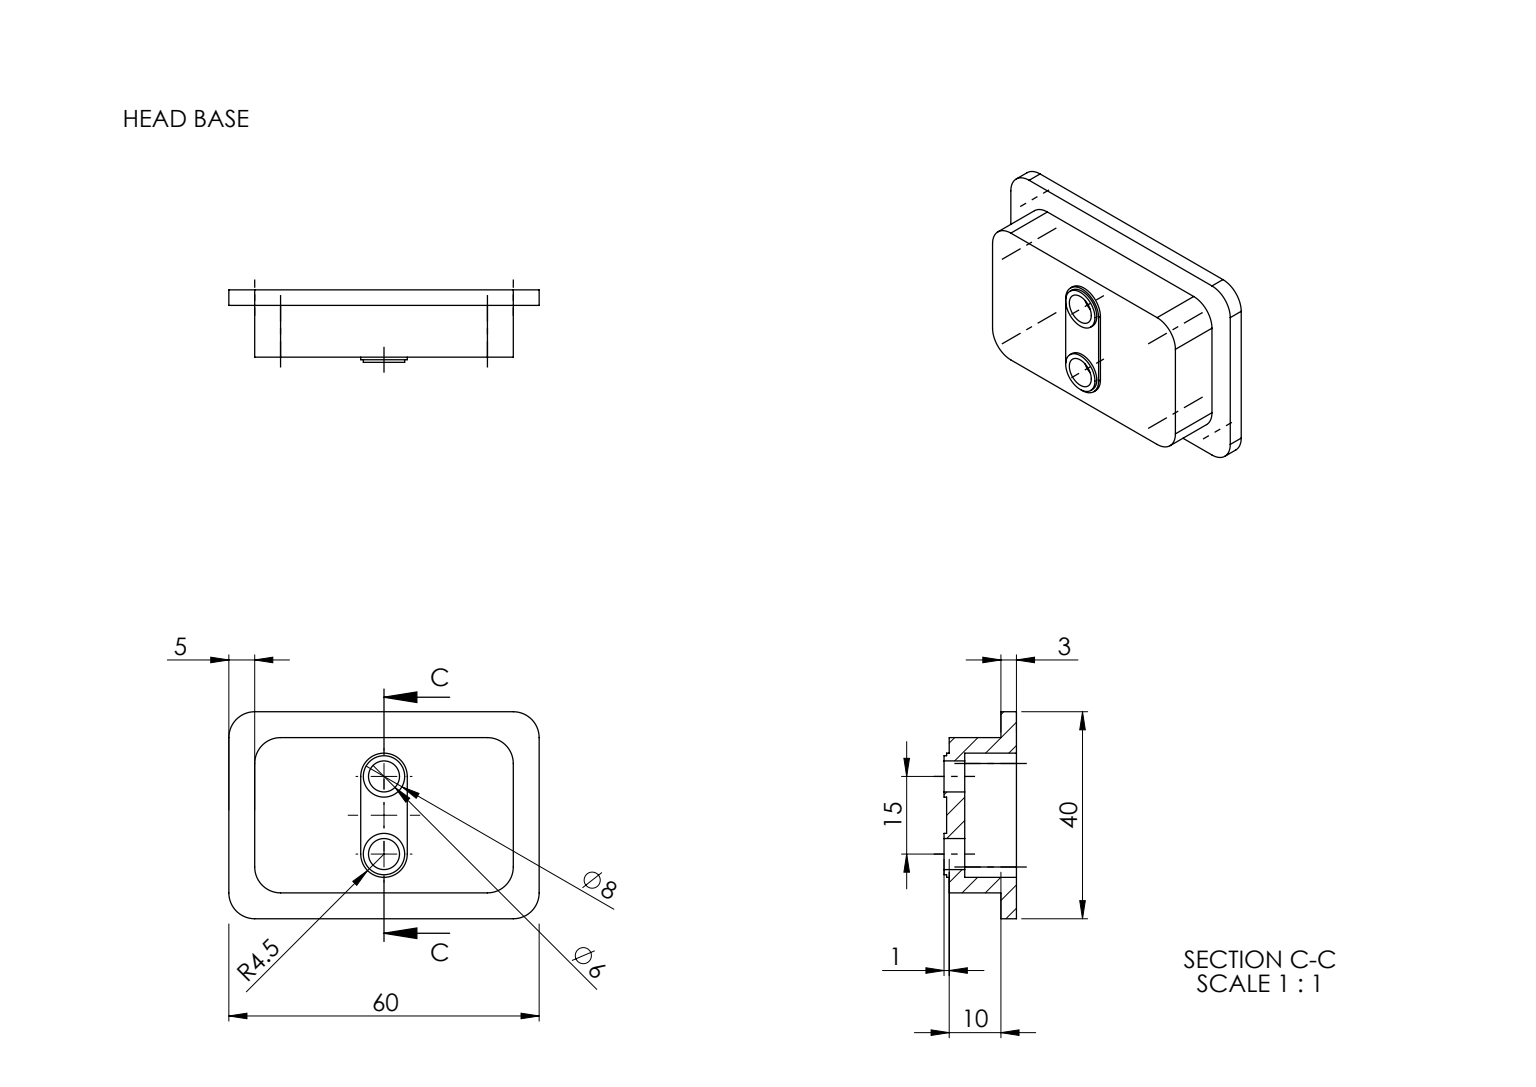
ISO-10303-21;
HEADER;
FILE_DESCRIPTION (('STEP AP214'),
    '1' );
FILE_NAME ('head base.step',
    '2026-10-05T05:16:24',
    ( '' ),
    ( '' ),
    'SwSTEP 2.0',
    'SolidWorks 2026',
    '' );
FILE_SCHEMA (( 'AUTOMOTIVE_DESIGN' ));
ENDSEC;

DATA;
#195=ORIENTED_EDGE ( 'NONE', *, *, #5496, .T. ) ;
#312=EDGE_CURVE ( 'NONE', #18504, #32170, #73011, .T. ) ;
#365=CARTESIAN_POINT ( 'NONE',  ( -19.99999999999996803, 12.00000000000000711, 13.00000000000000178 ) ) ;
#442=EDGE_CURVE ( 'NONE', #68729, #70011, #35447, .T. ) ;
#472=CARTESIAN_POINT ( 'NONE',  ( -19.99999999999996447, -15.00000000000000533, 13.00000000000000178 ) ) ;
#557=DIRECTION ( 'NONE',  ( -0.000000000000000000, -0.000000000000000000, 1.000000000000000000 ) ) ;
#647=ORIENTED_EDGE ( 'NONE', *, *, #5980, .F. ) ;
#855=FACE_OUTER_BOUND ( 'NONE', #52842, .T. ) ;
#984=EDGE_CURVE ( 'NONE', #16925, #51011, #66763, .T. ) ;
#1060=ORIENTED_EDGE ( 'NONE', *, *, #64186, .T. ) ;
#1108=VECTOR ( 'NONE', #67592, 1000.000000000000000 ) ;
#1176=CARTESIAN_POINT ( 'NONE',  ( -20.00000000000000355, 10.00000000000000711, 0.000000000000000000 ) ) ;
#1177=ORIENTED_EDGE ( 'NONE', *, *, #22871, .T. ) ;
#1205=EDGE_CURVE ( 'NONE', #18616, #63332, #75754, .T. ) ;
#1234=CARTESIAN_POINT ( 'NONE',  ( -30.00000000000000000, -15.00000000000000000, 0.000000000000000000 ) ) ;
#1306=EDGE_CURVE ( 'NONE', #63487, #26549, #52692, .T. ) ;
#1409=CARTESIAN_POINT ( 'NONE',  ( 1.653273178848927064E-15, -7.500000000000000000, 10.00000000000000178 ) ) ;
#1770=FACE_OUTER_BOUND ( 'NONE', #23896, .T. ) ;
#1802=EDGE_CURVE ( 'NONE', #18545, #32170, #34092, .T. ) ;
#2047=ORIENTED_EDGE ( 'NONE', *, *, #16725, .F. ) ;
#2074=EDGE_LOOP ( 'NONE', ( #21777, #5506, #55375, #74626, #78628, #49482, #5060, #5658 ) ) ;
#2087=EDGE_CURVE ( 'NONE', #19865, #25459, #46367, .T. ) ;
#2192=VERTEX_POINT ( 'NONE', #15248 ) ;
#2200=ORIENTED_EDGE ( 'NONE', *, *, #64434, .F. ) ;
#2202=DIRECTION ( 'NONE',  ( -1.000000000000000000, 0.000000000000000000, 0.000000000000000000 ) ) ;
#2315=VERTEX_POINT ( 'NONE', #64292 ) ;
#2378=DIRECTION ( 'NONE',  ( -1.000000000000000000, -0.000000000000000000, -0.000000000000000000 ) ) ;
#2534=CARTESIAN_POINT ( 'NONE',  ( 24.99999999999999645, -19.99999999999999645, 3.000000000000000000 ) ) ;
#2561=CARTESIAN_POINT ( 'NONE',  ( -2.939152317953646711E-15, 7.500000000000000000, 14.00000000000000178 ) ) ;
#2651=LINE ( 'NONE', #79222, #14432 ) ;
#2687=FACE_OUTER_BOUND ( 'NONE', #22273, .T. ) ;
#2987=DIRECTION ( 'NONE',  ( -0.000000000000000000, -0.000000000000000000, -1.000000000000000000 ) ) ;
#3039=ORIENTED_EDGE ( 'NONE', *, *, #49867, .T. ) ;
#3178=VECTOR ( 'NONE', #42643, 1000.000000000000000 ) ;
#3184=CARTESIAN_POINT ( 'NONE',  ( -4.000000000000002665, 7.500000000000000000, 14.00000000000000178 ) ) ;
#3289=ADVANCED_FACE ( 'NONE', ( #855 ), #21118, .F. ) ;
#3413=VERTEX_POINT ( 'NONE', #30098 ) ;
#3456=CARTESIAN_POINT ( 'NONE',  ( -24.99999999999999645, 20.00000000000000355, 3.000000000000000000 ) ) ;
#3577=LINE ( 'NONE', #17552, #29459 ) ;
#3768=EDGE_LOOP ( 'NONE', ( #32033, #51337, #64941, #21875 ) ) ;
#3841=FACE_OUTER_BOUND ( 'NONE', #46348, .T. ) ;
#4058=AXIS2_PLACEMENT_3D ( 'NONE', #29828, #76228, #28497 ) ;
#4063=EDGE_LOOP ( 'NONE', ( #83005, #56493, #12614, #77672 ) ) ;
#4204=DIRECTION ( 'NONE',  ( -1.000000000000000000, -2.602085213965214586E-16, 0.000000000000000000 ) ) ;
#4219=CIRCLE ( 'NONE', #9944, 2.000000000000001776 ) ;
#4406=AXIS2_PLACEMENT_3D ( 'NONE', #15425, #30695, #58160 ) ;
#4553=LINE ( 'NONE', #44629, #17255 ) ;
#4556=ORIENTED_EDGE ( 'NONE', *, *, #80069, .T. ) ;
#4604=CARTESIAN_POINT ( 'NONE',  ( 1.653273178848927064E-15, -7.500000000000000000, 14.00000000000000178 ) ) ;
#4629=FACE_OUTER_BOUND ( 'NONE', #4063, .T. ) ;
#4633=ADVANCED_FACE ( 'NONE', ( #24569 ), #63778, .T. ) ;
#4686=ADVANCED_FACE ( 'NONE', ( #25910 ), #17827, .F. ) ;
#4695=VERTEX_POINT ( 'NONE', #59692 ) ;
#4809=DIRECTION ( 'NONE',  ( 1.000000000000000000, 2.891205793294679312E-16, -0.000000000000000000 ) ) ;
#4928=AXIS2_PLACEMENT_3D ( 'NONE', #12936, #39980, #20576 ) ;
#4985=DIRECTION ( 'NONE',  ( -1.000000000000000000, 0.000000000000000000, 0.000000000000000000 ) ) ;
#5060=ORIENTED_EDGE ( 'NONE', *, *, #65557, .F. ) ;
#5101=LINE ( 'NONE', #66801, #28717 ) ;
#5110=VECTOR ( 'NONE', #83323, 1000.000000000000000 ) ;
#5172=VECTOR ( 'NONE', #59290, 1000.000000000000000 ) ;
#5413=EDGE_LOOP ( 'NONE', ( #8614, #19727 ) ) ;
#5496=EDGE_CURVE ( 'NONE', #18616, #70011, #21378, .T. ) ;
#5506=ORIENTED_EDGE ( 'NONE', *, *, #58155, .F. ) ;
#5519=ORIENTED_EDGE ( 'NONE', *, *, #46958, .F. ) ;
#5658=ORIENTED_EDGE ( 'NONE', *, *, #36655, .F. ) ;
#5674=( NAMED_UNIT ( * ) PLANE_ANGLE_UNIT ( ) SI_UNIT ( $, .RADIAN. ) );
#5765=CARTESIAN_POINT ( 'NONE',  ( 4.000000000000001776, -7.499999999999999112, 14.00000000000000178 ) ) ;
#5766=VERTEX_POINT ( 'NONE', #88001 ) ;
#5915=PRODUCT_CONTEXT ( 'NONE', #31413, 'mechanical' ) ;
#5969=DIRECTION ( 'NONE',  ( -1.000000000000000000, 0.000000000000000000, 0.000000000000000000 ) ) ;
#5980=EDGE_CURVE ( 'NONE', #81438, #38465, #26157, .T. ) ;
#6041=CARTESIAN_POINT ( 'NONE',  ( 22.00000000000000711, 9.999999999999971578, 10.00000000000000178 ) ) ;
#6065=CIRCLE ( 'NONE', #33378, 5.000000000000000888 ) ;
#6206=ORIENTED_EDGE ( 'NONE', *, *, #22249, .T. ) ;
#6220=ORIENTED_EDGE ( 'NONE', *, *, #1802, .T. ) ;
#6262=CARTESIAN_POINT ( 'NONE',  ( 25.00000000000000711, -9.999999999999957367, 3.000000000000000000 ) ) ;
#6281=LINE ( 'NONE', #81501, #58998 ) ;
#6523=CARTESIAN_POINT ( 'NONE',  ( 19.99999999999999289, -11.99999999999999467, 0.000000000000000000 ) ) ;
#6600=DIRECTION ( 'NONE',  ( -0.000000000000000000, -0.000000000000000000, 1.000000000000000000 ) ) ;
#6609=DIRECTION ( 'NONE',  ( 1.000000000000000000, 0.000000000000000000, 0.000000000000000000 ) ) ;
#6632=CARTESIAN_POINT ( 'NONE',  ( -25.00000000000000355, 9.999999999999971578, 3.000000000000000000 ) ) ;
#6641=ORIENTED_EDGE ( 'NONE', *, *, #16725, .T. ) ;
#6665=CIRCLE ( 'NONE', #57004, 5.000000000000000888 ) ;
#6846=EDGE_CURVE ( 'NONE', #66812, #61417, #24180, .T. ) ;
#6853=AXIS2_PLACEMENT_3D ( 'NONE', #39637, #81949, #32864 ) ;
#6906=DIRECTION ( 'NONE',  ( 1.734723475976812518E-16, -1.000000000000000000, 0.000000000000000000 ) ) ;
#6927=CARTESIAN_POINT ( 'NONE',  ( 20.00000000000000355, 10.00000000000000533, 13.00000000000000178 ) ) ;
#7173=DIRECTION ( 'NONE',  ( -0.000000000000000000, -0.000000000000000000, 1.000000000000000000 ) ) ;
#7184=CIRCLE ( 'NONE', #40303, 5.000000000000000888 ) ;
#7196=ORIENTED_EDGE ( 'NONE', *, *, #12757, .F. ) ;
#7303=EDGE_CURVE ( 'NONE', #16925, #38200, #58064, .T. ) ;
#7581=CARTESIAN_POINT ( 'NONE',  ( -2.939152317953646711E-15, 7.500000000000000000, 10.00000000000000178 ) ) ;
#7623=EDGE_CURVE ( 'NONE', #64470, #19590, #58845, .T. ) ;
#7645=EDGE_CURVE ( 'NONE', #69999, #32213, #86111, .T. ) ;
#7746=AXIS2_PLACEMENT_3D ( 'NONE', #88977, #53834, #14625 ) ;
#7760=FACE_OUTER_BOUND ( 'NONE', #35788, .T. ) ;
#7876=ORIENTED_EDGE ( 'NONE', *, *, #34261, .F. ) ;
#7893=ORIENTED_EDGE ( 'NONE', *, *, #21803, .F. ) ;
#7901=AXIS2_PLACEMENT_3D ( 'NONE', #17225, #51880, #38842 ) ;
#7983=ORIENTED_EDGE ( 'NONE', *, *, #56884, .F. ) ;
#8001=DIRECTION ( 'NONE',  ( -0.000000000000000000, -0.000000000000000000, -1.000000000000000000 ) ) ;
#8086=EDGE_CURVE ( 'NONE', #8684, #60639, #53111, .T. ) ;
#8216=ORIENTED_EDGE ( 'NONE', *, *, #51280, .F. ) ;
#8218=EDGE_CURVE ( 'NONE', #36898, #60372, #20437, .T. ) ;
#8277=LINE ( 'NONE', #56887, #35872 ) ;
#8309=VERTEX_POINT ( 'NONE', #69504 ) ;
#8320=DIRECTION ( 'NONE',  ( -0.000000000000000000, -0.000000000000000000, -1.000000000000000000 ) ) ;
#8330=ADVANCED_FACE ( 'NONE', ( #60368 ), #33352, .T. ) ;
#8402=VECTOR ( 'NONE', #71363, 1000.000000000000000 ) ;
#8408=DIRECTION ( 'NONE',  ( 1.000000000000000000, 0.000000000000000000, 0.000000000000000000 ) ) ;
#8537=AXIS2_PLACEMENT_3D ( 'NONE', #23795, #69789, #2202 ) ;
#8606=CIRCLE ( 'NONE', #58914, 4.500000000000001776 ) ;
#8614=ORIENTED_EDGE ( 'NONE', *, *, #76421, .F. ) ;
#8623=DIRECTION ( 'NONE',  ( 1.000000000000000000, 0.000000000000000000, 0.000000000000000000 ) ) ;
#8672=DIRECTION ( 'NONE',  ( 0.000000000000000000, 0.000000000000000000, 1.000000000000000000 ) ) ;
#8684=VERTEX_POINT ( 'NONE', #13111 ) ;
#8719=DIRECTION ( 'NONE',  ( 0.000000000000000000, 0.000000000000000000, 1.000000000000000000 ) ) ;
#8737=FACE_OUTER_BOUND ( 'NONE', #12896, .T. ) ;
#8784=AXIS2_PLACEMENT_3D ( 'NONE', #14973, #29817, #43326 ) ;
#8840=DIRECTION ( 'NONE',  ( -0.000000000000000000, -0.000000000000000000, -1.000000000000000000 ) ) ;
#8862=CARTESIAN_POINT ( 'NONE',  ( -30.00000000000000000, -15.00000000000000000, 3.000000000000000000 ) ) ;
#8964=EDGE_CURVE ( 'NONE', #8309, #60949, #86462, .T. ) ;
#9182=PRESENTATION_STYLE_ASSIGNMENT (( #42961 ) ) ;
#9211=CARTESIAN_POINT ( 'NONE',  ( -24.99999999999999645, -15.00000000000000000, 3.000000000000000000 ) ) ;
#9275=LINE ( 'NONE', #79051, #76492 ) ;
#9324=EDGE_CURVE ( 'NONE', #38200, #69999, #20864, .T. ) ;
#9651=VECTOR ( 'NONE', #77650, 1000.000000000000000 ) ;
#9660=EDGE_CURVE ( 'NONE', #30359, #38114, #86309, .T. ) ;
#9794=LINE ( 'NONE', #24640, #45704 ) ;
#9839=ADVANCED_FACE ( 'NONE', ( #2687, #15344 ), #42819, .T. ) ;
#9944=AXIS2_PLACEMENT_3D ( 'NONE', #70571, #83659, #76887 ) ;
#9994=AXIS2_PLACEMENT_3D ( 'NONE', #56497, #42983, #57818 ) ;
#10051=DIRECTION ( 'NONE',  ( 0.000000000000000000, 0.000000000000000000, 1.000000000000000000 ) ) ;
#10363=DIRECTION ( 'NONE',  ( -0.000000000000000000, -0.000000000000000000, -1.000000000000000000 ) ) ;
#10429=ORIENTED_EDGE ( 'NONE', *, *, #11533, .F. ) ;
#10541=AXIS2_PLACEMENT_3D ( 'NONE', #64258, #71913, #29614 ) ;
#10571=EDGE_CURVE ( 'NONE', #10700, #31320, #75066, .T. ) ;
#10596=CARTESIAN_POINT ( 'NONE',  ( 20.00000000000000711, -9.999999999999994671, 13.00000000000000178 ) ) ;
#10663=FILL_AREA_STYLE ('',( #72353 ) ) ;
#10700=VERTEX_POINT ( 'NONE', #85366 ) ;
#10748=ORIENTED_EDGE ( 'NONE', *, *, #18434, .T. ) ;
#10890=ORIENTED_EDGE ( 'NONE', *, *, #35603, .T. ) ;
#11062=ORIENTED_EDGE ( 'NONE', *, *, #24489, .F. ) ;
#11101=EDGE_LOOP ( 'NONE', ( #7876, #63098, #13245, #14650 ) ) ;
#11110=DIRECTION ( 'NONE',  ( 0.000000000000000000, 0.000000000000000000, 1.000000000000000000 ) ) ;
#11113=CARTESIAN_POINT ( 'NONE',  ( -2.939152317953646711E-15, 7.500000000000000000, 13.50000000000000178 ) ) ;
#11160=FACE_OUTER_BOUND ( 'NONE', #52351, .T. ) ;
#11256=LINE ( 'NONE', #59884, #79293 ) ;
#11358=PLANE ( 'NONE',  #7901 ) ;
#11403=ORIENTED_EDGE ( 'NONE', *, *, #67902, .T. ) ;
#11507=MECHANICAL_DESIGN_GEOMETRIC_PRESENTATION_REPRESENTATION('',(#14389),#21585);
#11533=EDGE_CURVE ( 'NONE', #68350, #38200, #11650, .T. ) ;
#11567=DIRECTION ( 'NONE',  ( 0.000000000000000000, 0.000000000000000000, 1.000000000000000000 ) ) ;
#11650=CIRCLE ( 'NONE', #83538, 2.000000000000001776 ) ;
#11703=EDGE_CURVE ( 'NONE', #32213, #60372, #13648, .T. ) ;
#11811=ORIENTED_EDGE ( 'NONE', *, *, #83550, .T. ) ;
#11889=ORIENTED_EDGE ( 'NONE', *, *, #9660, .T. ) ;
#11970=AXIS2_PLACEMENT_3D ( 'NONE', #40436, #48049, #8408 ) ;
#12354=PLANE ( 'NONE',  #13153 ) ;
#12436=CARTESIAN_POINT ( 'NONE',  ( -24.99999999999999645, 20.00000000000000355, 3.000000000000000000 ) ) ;
#12470=LINE ( 'NONE', #54330, #71773 ) ;
#12545=CARTESIAN_POINT ( 'NONE',  ( -24.99999999999999645, -19.99999999999999645, 0.000000000000000000 ) ) ;
#12614=ORIENTED_EDGE ( 'NONE', *, *, #23910, .F. ) ;
#12639=ORIENTED_EDGE ( 'NONE', *, *, #23910, .T. ) ;
#12694=ORIENTED_EDGE ( 'NONE', *, *, #19711, .T. ) ;
#12757=EDGE_CURVE ( 'NONE', #68985, #33215, #11256, .T. ) ;
#12830=ORIENTED_EDGE ( 'NONE', *, *, #84164, .F. ) ;
#12896=EDGE_LOOP ( 'NONE', ( #30436, #24948, #25039, #4556 ) ) ;
#12936=CARTESIAN_POINT ( 'NONE',  ( -24.99999999999999645, 15.00000000000000355, 3.000000000000000000 ) ) ;
#12944=FACE_OUTER_BOUND ( 'NONE', #69698, .T. ) ;
#13006=VECTOR ( 'NONE', #6600, 1000.000000000000000 ) ;
#13026=VECTOR ( 'NONE', #8001, 1000.000000000000000 ) ;
#13111=CARTESIAN_POINT ( 'NONE',  ( 24.99999999999999645, -19.99999999999999645, 0.000000000000000000 ) ) ;
#13129=CARTESIAN_POINT ( 'NONE',  ( -19.99999999999996803, 15.00000000000000711, 13.00000000000000178 ) ) ;
#13153=AXIS2_PLACEMENT_3D ( 'NONE', #59642, #53774, #87142 ) ;
#13231=VECTOR ( 'NONE', #19133, 1000.000000000000000 ) ;
#13245=ORIENTED_EDGE ( 'NONE', *, *, #13501, .T. ) ;
#13266=ORIENTED_EDGE ( 'NONE', *, *, #26362, .T. ) ;
#13271=CARTESIAN_POINT ( 'NONE',  ( 24.99999999999999645, -19.99999999999999645, 3.000000000000000000 ) ) ;
#13338=AXIS2_PLACEMENT_3D ( 'NONE', #365, #61609, #40908 ) ;
#13429=PLANE ( 'NONE',  #13338 ) ;
#13501=EDGE_CURVE ( 'NONE', #36898, #71705, #47720, .T. ) ;
#13528=VECTOR ( 'NONE', #71559, 1000.000000000000000 ) ;
#13638=CARTESIAN_POINT ( 'NONE',  ( 30.00000000000000000, 15.00000000000000355, 0.000000000000000000 ) ) ;
#13648=LINE ( 'NONE', #75789, #23148 ) ;
#13663=CARTESIAN_POINT ( 'NONE',  ( 3.000000000000001776, -7.500000000000000000, 0.000000000000000000 ) ) ;
#13752=LINE ( 'NONE', #53403, #13995 ) ;
#13768=CIRCLE ( 'NONE', #87166, 3.000000000000000444 ) ;
#13959=FACE_OUTER_BOUND ( 'NONE', #83885, .T. ) ;
#13995=VECTOR ( 'NONE', #20073, 1000.000000000000000 ) ;
#14051=ORIENTED_EDGE ( 'NONE', *, *, #5980, .T. ) ;
#14083=EDGE_CURVE ( 'NONE', #60639, #81205, #64753, .T. ) ;
#14126=EDGE_LOOP ( 'NONE', ( #30032, #47464, #76118, #83266 ) ) ;
#14164=AXIS2_PLACEMENT_3D ( 'NONE', #36806, #11110, #86352 ) ;
#14205=VERTEX_POINT ( 'NONE', #59789 ) ;
#14361=CARTESIAN_POINT ( 'NONE',  ( -22.00000000000000711, 9.999999999999971578, 0.000000000000000000 ) ) ;
#14389=STYLED_ITEM ( 'NONE', ( #9182 ), #73996 ) ;
#14432=VECTOR ( 'NONE', #60271, 1000.000000000000000 ) ;
#14572=ADVANCED_FACE ( 'NONE', ( #4629 ), #53249, .F. ) ;
#14604=EDGE_CURVE ( 'NONE', #51011, #17681, #57730, .T. ) ;
#14625=DIRECTION ( 'NONE',  ( 1.000000000000000000, 0.000000000000000000, -0.000000000000000000 ) ) ;
#14650=ORIENTED_EDGE ( 'NONE', *, *, #20454, .T. ) ;
#14708=DIRECTION ( 'NONE',  ( -0.000000000000000000, -0.000000000000000000, -1.000000000000000000 ) ) ;
#14744=ORIENTED_EDGE ( 'NONE', *, *, #70435, .T. ) ;
#14937=ORIENTED_EDGE ( 'NONE', *, *, #40107, .F. ) ;
#14973=CARTESIAN_POINT ( 'NONE',  ( 1.653273178848927064E-15, -7.500000000000000000, 14.00000000000000178 ) ) ;
#15066=ORIENTED_EDGE ( 'NONE', *, *, #60476, .F. ) ;
#15146=DIRECTION ( 'NONE',  ( 0.000000000000000000, 0.000000000000000000, 1.000000000000000000 ) ) ;
#15170=LINE ( 'NONE', #34986, #3178 ) ;
#15187=DIRECTION ( 'NONE',  ( -0.000000000000000000, -0.000000000000000000, -1.000000000000000000 ) ) ;
#15248=CARTESIAN_POINT ( 'NONE',  ( 19.99999999999996803, 12.00000000000000711, 10.00000000000000178 ) ) ;
#15344=FACE_BOUND ( 'NONE', #68935, .T. ) ;
#15377=AXIS2_PLACEMENT_3D ( 'NONE', #36820, #85019, #77366 ) ;
#15394=EDGE_LOOP ( 'NONE', ( #27022, #12830, #647, #52526 ) ) ;
#15419=FACE_BOUND ( 'NONE', #79429, .T. ) ;
#15425=CARTESIAN_POINT ( 'NONE',  ( 24.99999999999999645, 15.00000000000000355, 0.000000000000000000 ) ) ;
#15476=CARTESIAN_POINT ( 'NONE',  ( -24.99999999999999645, -15.00000000000000000, 0.000000000000000000 ) ) ;
#15490=SHAPE_REPRESENTATION_RELATIONSHIP ( 'NONE' , 'NONE' ,  #85713, #73996 ) ;
#15496=CARTESIAN_POINT ( 'NONE',  ( 1.653273178848927064E-15, -7.500000000000000000, 10.00000000000000178 ) ) ;
#15556=AXIS2_PLACEMENT_3D ( 'NONE', #57893, #17359, #70974 ) ;
#15637=VECTOR ( 'NONE', #45329, 1000.000000000000000 ) ;
#15638=ORIENTED_EDGE ( 'NONE', *, *, #83550, .F. ) ;
#15649=VERTEX_POINT ( 'NONE', #21728 ) ;
#15667=LINE ( 'NONE', #43137, #86476 ) ;
#15953=VECTOR ( 'NONE', #78730, 1000.000000000000000 ) ;
#16150=ORIENTED_EDGE ( 'NONE', *, *, #36183, .T. ) ;
#16324=CARTESIAN_POINT ( 'NONE',  ( 22.00000000000000711, 9.999999999999991118, 10.00000000000000178 ) ) ;
#16369=ORIENTED_EDGE ( 'NONE', *, *, #81297, .F. ) ;
#16389=PLANE ( 'NONE',  #38761 ) ;
#16399=ORIENTED_EDGE ( 'NONE', *, *, #78408, .F. ) ;
#16438=LINE ( 'NONE', #43907, #32432 ) ;
#16487=DIRECTION ( 'NONE',  ( -0.000000000000000000, -0.000000000000000000, -1.000000000000000000 ) ) ;
#16528=DIRECTION ( 'NONE',  ( 1.000000000000000000, 0.000000000000000000, 0.000000000000000000 ) ) ;
#16641=DIRECTION ( 'NONE',  ( 0.000000000000000000, 0.000000000000000000, 1.000000000000000000 ) ) ;
#16725=EDGE_CURVE ( 'NONE', #31293, #17102, #6065, .T. ) ;
#16783=DIRECTION ( 'NONE',  ( -1.000000000000000000, 0.000000000000000000, 0.000000000000000000 ) ) ;
#16805=VECTOR ( 'NONE', #67005, 1000.000000000000000 ) ;
#16889=VECTOR ( 'NONE', #87328, 1000.000000000000000 ) ;
#16900=DIRECTION ( 'NONE',  ( 1.000000000000000000, 0.000000000000000000, 0.000000000000000000 ) ) ;
#16925=VERTEX_POINT ( 'NONE', #23400 ) ;
#17037=ADVANCED_FACE ( 'NONE', ( #71148 ), #36917, .T. ) ;
#17051=VERTEX_POINT ( 'NONE', #34162 ) ;
#17093=EDGE_LOOP ( 'NONE', ( #83307, #21231, #88931, #17741 ) ) ;
#17102=VERTEX_POINT ( 'NONE', #6262 ) ;
#17111=CARTESIAN_POINT ( 'NONE',  ( -30.00000000000000000, 15.00000000000000355, 3.000000000000000000 ) ) ;
#17223=CARTESIAN_POINT ( 'NONE',  ( 1.653273178848927064E-15, -7.500000000000000000, 14.00000000000000178 ) ) ;
#17225=CARTESIAN_POINT ( 'NONE',  ( 4.499999999999999112, 7.500000000000002665, 13.50000000000000178 ) ) ;
#17229=DIRECTION ( 'NONE',  ( -1.000000000000000000, 0.000000000000000000, 0.000000000000000000 ) ) ;
#17255=VECTOR ( 'NONE', #24817, 1000.000000000000000 ) ;
#17344=CARTESIAN_POINT ( 'NONE',  ( -20.00000000000000355, -10.00000000000000533, 13.00000000000000178 ) ) ;
#17359=DIRECTION ( 'NONE',  ( -0.000000000000000000, -0.000000000000000000, -1.000000000000000000 ) ) ;
#17388=CIRCLE ( 'NONE', #46147, 5.000000000000000888 ) ;
#17524=FACE_BOUND ( 'NONE', #79964, .T. ) ;
#17552=CARTESIAN_POINT ( 'NONE',  ( 4.499999999999999112, 7.500000000000002665, 13.50000000000000178 ) ) ;
#17662=CARTESIAN_POINT ( 'NONE',  ( -30.00000000000000000, 15.00000000000000355, 3.000000000000000000 ) ) ;
#17681=VERTEX_POINT ( 'NONE', #65063 ) ;
#17741=ORIENTED_EDGE ( 'NONE', *, *, #21803, .T. ) ;
#17827=PLANE ( 'NONE',  #28511 ) ;
#17868=DIRECTION ( 'NONE',  ( 0.000000000000000000, 0.000000000000000000, 1.000000000000000000 ) ) ;
#17953=EDGE_LOOP ( 'NONE', ( #74100, #62548, #41992, #41745 ) ) ;
#17976=ORIENTED_EDGE ( 'NONE', *, *, #44356, .F. ) ;
#18066=EDGE_CURVE ( 'NONE', #40270, #61417, #25208, .T. ) ;
#18115=CARTESIAN_POINT ( 'NONE',  ( 19.99999999999999289, -11.99999999999999467, 10.00000000000000178 ) ) ;
#18149=CARTESIAN_POINT ( 'NONE',  ( 30.00000000000000000, -15.00000000000000000, 3.000000000000000000 ) ) ;
#18192=DIRECTION ( 'NONE',  ( 0.000000000000000000, 0.000000000000000000, 1.000000000000000000 ) ) ;
#18434=EDGE_CURVE ( 'NONE', #73496, #15649, #31557, .T. ) ;
#18466=EDGE_CURVE ( 'NONE', #59616, #19865, #46490, .T. ) ;
#18504=VERTEX_POINT ( 'NONE', #61566 ) ;
#18530=EDGE_CURVE ( 'NONE', #22067, #22580, #49391, .T. ) ;
#18545=VERTEX_POINT ( 'NONE', #48941 ) ;
#18616=VERTEX_POINT ( 'NONE', #57021 ) ;
#18653=LINE ( 'NONE', #59620, #76335 ) ;
#18674=FACE_OUTER_BOUND ( 'NONE', #2074, .T. ) ;
#18826=VERTEX_POINT ( 'NONE', #19157 ) ;
#18855=PLANE ( 'NONE',  #26581 ) ;
#18919=DIRECTION ( 'NONE',  ( -2.891205793294678326E-16, 1.000000000000000000, -0.000000000000000000 ) ) ;
#19056=ORIENTED_EDGE ( 'NONE', *, *, #26362, .F. ) ;
#19133=DIRECTION ( 'NONE',  ( -0.000000000000000000, -0.000000000000000000, -1.000000000000000000 ) ) ;
#19157=CARTESIAN_POINT ( 'NONE',  ( 30.00000000000000000, -15.00000000000000000, 3.000000000000000000 ) ) ;
#19175=EDGE_LOOP ( 'NONE', ( #34540, #16399, #80837, #56876 ) ) ;
#19177=ORIENTED_EDGE ( 'NONE', *, *, #75759, .T. ) ;
#19407=CIRCLE ( 'NONE', #88419, 3.000000000000000000 ) ;
#19474=DIRECTION ( 'NONE',  ( -0.000000000000000000, -0.000000000000000000, -1.000000000000000000 ) ) ;
#19503=FACE_OUTER_BOUND ( 'NONE', #73049, .T. ) ;
#19558=ORIENTED_EDGE ( 'NONE', *, *, #38282, .T. ) ;
#19590=VERTEX_POINT ( 'NONE', #36443 ) ;
#19606=FACE_OUTER_BOUND ( 'NONE', #49192, .T. ) ;
#19664=DIRECTION ( 'NONE',  ( 0.000000000000000000, 1.000000000000000000, 0.000000000000000000 ) ) ;
#19711=EDGE_CURVE ( 'NONE', #4695, #17051, #78748, .T. ) ;
#19727=ORIENTED_EDGE ( 'NONE', *, *, #36136, .F. ) ;
#19757=CARTESIAN_POINT ( 'NONE',  ( -24.99999999999999645, -19.99999999999999645, 3.000000000000000000 ) ) ;
#19865=VERTEX_POINT ( 'NONE', #5765 ) ;
#19892=ORIENTED_EDGE ( 'NONE', *, *, #42792, .T. ) ;
#19919=ORIENTED_EDGE ( 'NONE', *, *, #9324, .T. ) ;
#19944=ORIENTED_EDGE ( 'NONE', *, *, #62373, .F. ) ;
#20073=DIRECTION ( 'NONE',  ( -0.000000000000000000, -0.000000000000000000, -1.000000000000000000 ) ) ;
#20238=CIRCLE ( 'NONE', #4406, 5.000000000000000888 ) ;
#20400=VERTEX_POINT ( 'NONE', #31119 ) ;
#20413=DIRECTION ( 'NONE',  ( 0.000000000000000000, 0.000000000000000000, 1.000000000000000000 ) ) ;
#20437=LINE ( 'NONE', #40720, #48737 ) ;
#20454=EDGE_CURVE ( 'NONE', #71705, #22195, #74345, .T. ) ;
#20468=ORIENTED_EDGE ( 'NONE', *, *, #29865, .T. ) ;
#20576=DIRECTION ( 'NONE',  ( -1.000000000000000000, 0.000000000000000000, 0.000000000000000000 ) ) ;
#20587=ORIENTED_EDGE ( 'NONE', *, *, #46958, .T. ) ;
#20594=AXIS2_PLACEMENT_3D ( 'NONE', #56188, #17868, #39480 ) ;
#20864=LINE ( 'NONE', #34378, #48810 ) ;
#20928=FACE_BOUND ( 'NONE', #69239, .T. ) ;
#21028=EDGE_LOOP ( 'NONE', ( #31715, #28055, #61276, #11403 ) ) ;
#21031=CARTESIAN_POINT ( 'NONE',  ( -2.939152317953646711E-15, 7.500000000000000000, 14.00000000000000178 ) ) ;
#21077=DIRECTION ( 'NONE',  ( 1.000000000000000000, 0.000000000000000000, 0.000000000000000000 ) ) ;
#21118=CYLINDRICAL_SURFACE ( 'NONE', #68762, 3.000000000000000444 ) ;
#21231=ORIENTED_EDGE ( 'NONE', *, *, #80069, .F. ) ;
#21358=ORIENTED_EDGE ( 'NONE', *, *, #54212, .T. ) ;
#21371=ORIENTED_EDGE ( 'NONE', *, *, #8964, .T. ) ;
#21378=LINE ( 'NONE', #50161, #9651 ) ;
#21386=AXIS2_PLACEMENT_3D ( 'NONE', #8862, #56154, #63348 ) ;
#21552=AXIS2_PLACEMENT_3D ( 'NONE', #74381, #72595, #46464 ) ;
#21585=( GEOMETRIC_REPRESENTATION_CONTEXT ( 3 ) GLOBAL_UNCERTAINTY_ASSIGNED_CONTEXT ( ( #23001 ) ) GLOBAL_UNIT_ASSIGNED_CONTEXT ( ( #49270, #56469, #71296 ) ) REPRESENTATION_CONTEXT ( 'NONE', 'WORKASPACE' ) );
#21708=ORIENTED_EDGE ( 'NONE', *, *, #36136, .T. ) ;
#21728=CARTESIAN_POINT ( 'NONE',  ( 2.999999999999997335, 7.500000000000000000, 14.00000000000000178 ) ) ;
#21737=CARTESIAN_POINT ( 'NONE',  ( -25.00000000000000355, 9.999999999999971578, 3.000000000000000000 ) ) ;
#21777=ORIENTED_EDGE ( 'NONE', *, *, #13501, .F. ) ;
#21803=EDGE_CURVE ( 'NONE', #17681, #32213, #23708, .T. ) ;
#21824=VECTOR ( 'NONE', #56952, 1000.000000000000000 ) ;
#21827=CYLINDRICAL_SURFACE ( 'NONE', #68239, 5.000000000000000888 ) ;
#21857=CARTESIAN_POINT ( 'NONE',  ( -25.00000000000000355, 9.999999999999971578, 13.00000000000000178 ) ) ;
#21875=ORIENTED_EDGE ( 'NONE', *, *, #41723, .T. ) ;
#21950=ORIENTED_EDGE ( 'NONE', *, *, #22509, .F. ) ;
#21964=FACE_BOUND ( 'NONE', #79199, .T. ) ;
#22067=VERTEX_POINT ( 'NONE', #21737 ) ;
#22195=VERTEX_POINT ( 'NONE', #23937 ) ;
#22215=ORIENTED_EDGE ( 'NONE', *, *, #77394, .T. ) ;
#22249=EDGE_CURVE ( 'NONE', #32170, #79550, #81574, .T. ) ;
#22263=ADVANCED_FACE ( 'NONE', ( #32938 ), #60844, .F. ) ;
#22273=EDGE_LOOP ( 'NONE', ( #11062, #19944, #52099, #21950, #16369, #27894, #86581, #74895 ) ) ;
#22401=PLANE ( 'NONE',  #59441 ) ;
#22498=LINE ( 'NONE', #58047, #13528 ) ;
#22509=EDGE_CURVE ( 'NONE', #50943, #66812, #86912, .T. ) ;
#22580=VERTEX_POINT ( 'NONE', #39157 ) ;
#22694=CARTESIAN_POINT ( 'NONE',  ( 19.99999999999997158, -14.99999999999999467, 3.000000000000000000 ) ) ;
#22697=VECTOR ( 'NONE', #68168, 1000.000000000000000 ) ;
#22744=LINE ( 'NONE', #50204, #56420 ) ;
#22769=VECTOR ( 'NONE', #45437, 1000.000000000000000 ) ;
#22857=DIRECTION ( 'NONE',  ( 1.000000000000000000, 2.602085213965214586E-16, 0.000000000000000000 ) ) ;
#22863=VECTOR ( 'NONE', #15187, 1000.000000000000000 ) ;
#22871=EDGE_CURVE ( 'NONE', #85628, #8309, #8606, .T. ) ;
#22894=CARTESIAN_POINT ( 'NONE',  ( 30.00000000000000000, -15.00000000000000000, 0.000000000000000000 ) ) ;
#23001=UNCERTAINTY_MEASURE_WITH_UNIT (LENGTH_MEASURE( 1.000000000000000082E-05 ), #49270, 'distance_accuracy_value', 'NONE');
#23051=PRODUCT_DEFINITION_CONTEXT ( 'detailed design', #88395, 'design' ) ;
#23148=VECTOR ( 'NONE', #33484, 1000.000000000000000 ) ;
#23274=EDGE_CURVE ( 'NONE', #79550, #22067, #7184, .T. ) ;
#23400=CARTESIAN_POINT ( 'NONE',  ( -22.00000000000000711, 9.999999999999971578, 10.00000000000000178 ) ) ;
#23427=MECHANICAL_DESIGN_GEOMETRIC_PRESENTATION_REPRESENTATION('',(#63737),#55130);
#23608=CARTESIAN_POINT ( 'NONE',  ( 30.00000000000000000, 15.00000000000000355, 3.000000000000000000 ) ) ;
#23653=DIRECTION ( 'NONE',  ( -1.000000000000000000, 0.000000000000000000, 0.000000000000000000 ) ) ;
#23655=CARTESIAN_POINT ( 'NONE',  ( -22.00000000000000355, -10.00000000000000533, 0.000000000000000000 ) ) ;
#23708=LINE ( 'NONE', #36794, #68495 ) ;
#23733=VECTOR ( 'NONE', #34844, 1000.000000000000000 ) ;
#23749=DIRECTION ( 'NONE',  ( -1.734723475976813504E-16, 1.000000000000000000, 0.000000000000000000 ) ) ;
#23795=CARTESIAN_POINT ( 'NONE',  ( -2.939152317953646711E-15, 7.500000000000000000, 14.00000000000000178 ) ) ;
#23800=ORIENTED_EDGE ( 'NONE', *, *, #7645, .T. ) ;
#23896=EDGE_LOOP ( 'NONE', ( #31891, #88365, #42732, #62617 ) ) ;
#23910=EDGE_CURVE ( 'NONE', #18826, #84614, #40396, .T. ) ;
#23923=ORIENTED_EDGE ( 'NONE', *, *, #22509, .T. ) ;
#23924=VECTOR ( 'NONE', #87504, 1000.000000000000000 ) ;
#23937=CARTESIAN_POINT ( 'NONE',  ( 22.00000000000001066, -9.999999999999957367, 0.000000000000000000 ) ) ;
#23952=EDGE_LOOP ( 'NONE', ( #11889, #71790 ) ) ;
#24007=ORIENTED_EDGE ( 'NONE', *, *, #27409, .T. ) ;
#24032=CARTESIAN_POINT ( 'NONE',  ( -3.999999999999998224, -7.500000000000000000, 14.00000000000000178 ) ) ;
#24149=ADVANCED_FACE ( 'NONE', ( #37163 ), #30415, .F. ) ;
#24180=CIRCLE ( 'NONE', #4058, 5.000000000000000888 ) ;
#24197=PLANE ( 'NONE',  #45421 ) ;
#24232=ORIENTED_EDGE ( 'NONE', *, *, #18530, .T. ) ;
#24294=EDGE_LOOP ( 'NONE', ( #19892, #19177, #52080, #77758, #41495, #12694, #86417, #14051 ) ) ;
#24403=DIRECTION ( 'NONE',  ( -0.000000000000000000, -0.000000000000000000, -1.000000000000000000 ) ) ;
#24419=FACE_OUTER_BOUND ( 'NONE', #40427, .T. ) ;
#24462=VECTOR ( 'NONE', #71501, 1000.000000000000000 ) ;
#24489=EDGE_CURVE ( 'NONE', #34053, #34010, #17388, .T. ) ;
#24492=CARTESIAN_POINT ( 'NONE',  ( -2.939152317953646711E-15, 7.500000000000000000, 14.00000000000000178 ) ) ;
#24569=FACE_OUTER_BOUND ( 'NONE', #74667, .T. ) ;
#24640=CARTESIAN_POINT ( 'NONE',  ( 4.499999999999999112, 7.500000000000002665, 13.50000000000000178 ) ) ;
#24711=CARTESIAN_POINT ( 'NONE',  ( 25.00000000000000355, 9.999999999999971578, 13.00000000000000178 ) ) ;
#24724=ORIENTED_EDGE ( 'NONE', *, *, #49596, .F. ) ;
#24761=CARTESIAN_POINT ( 'NONE',  ( 4.000000000000001776, -7.499999999999999112, 14.00000000000000178 ) ) ;
#24795=DIRECTION ( 'NONE',  ( -0.000000000000000000, -0.000000000000000000, 1.000000000000000000 ) ) ;
#24800=ORIENTED_EDGE ( 'NONE', *, *, #85079, .F. ) ;
#24817=DIRECTION ( 'NONE',  ( -0.000000000000000000, -0.000000000000000000, -1.000000000000000000 ) ) ;
#24871=CARTESIAN_POINT ( 'NONE',  ( 25.00000000000000355, 9.999999999999971578, 3.000000000000000000 ) ) ;
#24876=VECTOR ( 'NONE', #10363, 1000.000000000000000 ) ;
#24902=AXIS2_PLACEMENT_3D ( 'NONE', #12436, #39921, #74585 ) ;
#24941=ORIENTED_EDGE ( 'NONE', *, *, #24489, .T. ) ;
#24948=ORIENTED_EDGE ( 'NONE', *, *, #7303, .F. ) ;
#25039=ORIENTED_EDGE ( 'NONE', *, *, #984, .T. ) ;
#25066=CYLINDRICAL_SURFACE ( 'NONE', #68903, 3.000000000000000000 ) ;
#25102=CIRCLE ( 'NONE', #65340, 5.000000000000000888 ) ;
#25134=DIRECTION ( 'NONE',  ( -1.000000000000000000, 0.000000000000000000, 0.000000000000000000 ) ) ;
#25187=ORIENTED_EDGE ( 'NONE', *, *, #18434, .F. ) ;
#25208=LINE ( 'NONE', #17111, #24876 ) ;
#25250=ADVANCED_FACE ( 'NONE', ( #19503, #15419 ), #56831, .T. ) ;
#25420=FACE_BOUND ( 'NONE', #77321, .T. ) ;
#25423=DIRECTION ( 'NONE',  ( 1.000000000000000000, 0.000000000000000000, 0.000000000000000000 ) ) ;
#25446=LINE ( 'NONE', #73191, #13231 ) ;
#25459=VERTEX_POINT ( 'NONE', #52732 ) ;
#25474=CIRCLE ( 'NONE', #87345, 3.000000000000000444 ) ;
#25534=CARTESIAN_POINT ( 'NONE',  ( -19.99999999999998934, 12.00000000000000711, 0.000000000000000000 ) ) ;
#25593=EDGE_LOOP ( 'NONE', ( #65987, #40287, #8216, #59914 ) ) ;
#25755=DIRECTION ( 'NONE',  ( 0.000000000000000000, -0.000000000000000000, -1.000000000000000000 ) ) ;
#25792=CARTESIAN_POINT ( 'NONE',  ( -20.00000000000000355, -10.00000000000000533, 10.00000000000000178 ) ) ;
#25869=DIRECTION ( 'NONE',  ( 0.000000000000000000, 0.000000000000000000, 1.000000000000000000 ) ) ;
#25910=FACE_OUTER_BOUND ( 'NONE', #14126, .T. ) ;
#26046=AXIS2_PLACEMENT_3D ( 'NONE', #79850, #5969, #87973 ) ;
#26157=LINE ( 'NONE', #60379, #1108 ) ;
#26362=EDGE_CURVE ( 'NONE', #40270, #33584, #87225, .T. ) ;
#26549=VERTEX_POINT ( 'NONE', #59176 ) ;
#26581=AXIS2_PLACEMENT_3D ( 'NONE', #59835, #60723, #81011 ) ;
#26585=ORIENTED_EDGE ( 'NONE', *, *, #11533, .T. ) ;
#26789=ORIENTED_EDGE ( 'NONE', *, *, #36183, .F. ) ;
#26808=EDGE_CURVE ( 'NONE', #20400, #16925, #69348, .T. ) ;
#27022=ORIENTED_EDGE ( 'NONE', *, *, #40973, .T. ) ;
#27400=DIRECTION ( 'NONE',  ( -0.000000000000000000, -0.000000000000000000, -1.000000000000000000 ) ) ;
#27409=EDGE_CURVE ( 'NONE', #2192, #20400, #22744, .T. ) ;
#27496=AXIS2_PLACEMENT_3D ( 'NONE', #7581, #62940, #21077 ) ;
#27514=DIRECTION ( 'NONE',  ( 0.000000000000000000, 0.000000000000000000, 1.000000000000000000 ) ) ;
#27557=ORIENTED_EDGE ( 'NONE', *, *, #53279, .F. ) ;
#27629=LINE ( 'NONE', #6041, #84319 ) ;
#27648=CARTESIAN_POINT ( 'NONE',  ( -30.00000000000000000, -15.00000000000000000, 0.000000000000000000 ) ) ;
#27672=ORIENTED_EDGE ( 'NONE', *, *, #6846, .T. ) ;
#27688=CARTESIAN_POINT ( 'NONE',  ( 22.00000000000000711, 9.999999999999991118, 0.000000000000000000 ) ) ;
#27715=EDGE_CURVE ( 'NONE', #37043, #5766, #70886, .T. ) ;
#27828=FACE_OUTER_BOUND ( 'NONE', #50215, .T. ) ;
#27894=ORIENTED_EDGE ( 'NONE', *, *, #14083, .F. ) ;
#28043=CARTESIAN_POINT ( 'NONE',  ( -20.00000000000000355, -10.00000000000000533, 13.00000000000000178 ) ) ;
#28055=ORIENTED_EDGE ( 'NONE', *, *, #60734, .F. ) ;
#28088=ORIENTED_EDGE ( 'NONE', *, *, #312, .F. ) ;
#28094=LINE ( 'NONE', #27648, #23733 ) ;
#28249=ADVANCED_FACE ( 'NONE', ( #27828 ), #13429, .T. ) ;
#28310=ADVANCED_FACE ( 'NONE', ( #83679, #21964 ), #22401, .F. ) ;
#28372=EDGE_CURVE ( 'NONE', #5766, #37043, #32114, .T. ) ;
#28373=VECTOR ( 'NONE', #73851, 1000.000000000000000 ) ;
#28450=MANIFOLD_SOLID_BREP ( 'Boss-Extrude3', #78941 ) ;
#28473=AXIS2_PLACEMENT_3D ( 'NONE', #55907, #76181, #62657 ) ;
#28497=DIRECTION ( 'NONE',  ( -1.000000000000000000, 0.000000000000000000, 0.000000000000000000 ) ) ;
#28508=ADVANCED_FACE ( 'NONE', ( #55626 ), #83116, .F. ) ;
#28511=AXIS2_PLACEMENT_3D ( 'NONE', #66453, #31785, #32228 ) ;
#28610=CARTESIAN_POINT ( 'NONE',  ( -30.00000000000000000, -15.00000000000000000, 3.000000000000000000 ) ) ;
#28717=VECTOR ( 'NONE', #39784, 1000.000000000000000 ) ;
#29022=DIRECTION ( 'NONE',  ( 1.000000000000000000, 0.000000000000000000, 0.000000000000000000 ) ) ;
#29113=AXIS2_PLACEMENT_3D ( 'NONE', #44101, #16641, #71581 ) ;
#29241=CARTESIAN_POINT ( 'NONE',  ( -20.00000000000000355, 10.00000000000000711, 13.00000000000000178 ) ) ;
#29347=DIRECTION ( 'NONE',  ( -0.000000000000000000, -0.000000000000000000, -1.000000000000000000 ) ) ;
#29386=CIRCLE ( 'NONE', #58159, 5.000000000000000888 ) ;
#29459=VECTOR ( 'NONE', #79252, 1000.000000000000000 ) ;
#29536=CARTESIAN_POINT ( 'NONE',  ( -20.00000000000000355, 10.00000000000000711, 13.00000000000000178 ) ) ;
#29604=DIRECTION ( 'NONE',  ( -1.000000000000000000, 0.000000000000000000, 0.000000000000000000 ) ) ;
#29614=DIRECTION ( 'NONE',  ( 1.000000000000000000, 0.000000000000000000, 0.000000000000000000 ) ) ;
#29651=ADVANCED_FACE ( 'NONE', ( #11160 ), #80520, .F. ) ;
#29654=ORIENTED_EDGE ( 'NONE', *, *, #74036, .F. ) ;
#29696=CYLINDRICAL_SURFACE ( 'NONE', #8537, 4.000000000000000000 ) ;
#29774=DIRECTION ( 'NONE',  ( 0.000000000000000000, 0.000000000000000000, 1.000000000000000000 ) ) ;
#29817=DIRECTION ( 'NONE',  ( 0.000000000000000000, 0.000000000000000000, 1.000000000000000000 ) ) ;
#29828=CARTESIAN_POINT ( 'NONE',  ( -24.99999999999999645, 15.00000000000000355, 0.000000000000000000 ) ) ;
#29865=EDGE_CURVE ( 'NONE', #19590, #40270, #43741, .T. ) ;
#29898=CIRCLE ( 'NONE', #28473, 4.000000000000000000 ) ;
#29916=DIRECTION ( 'NONE',  ( -2.602085213965214586E-16, 1.000000000000000000, 0.000000000000000000 ) ) ;
#30007=AXIS2_PLACEMENT_3D ( 'NONE', #66682, #39671, #4985 ) ;
#30031=CYLINDRICAL_SURFACE ( 'NONE', #88237, 4.999999999999997335 ) ;
#30032=ORIENTED_EDGE ( 'NONE', *, *, #42626, .T. ) ;
#30086=CARTESIAN_POINT ( 'NONE',  ( 25.00000000000000711, -9.999999999999957367, 13.00000000000000178 ) ) ;
#30098=CARTESIAN_POINT ( 'NONE',  ( -24.99999999999999645, -19.99999999999999645, 3.000000000000000000 ) ) ;
#30110=EDGE_CURVE ( 'NONE', #18826, #60639, #31662, .T. ) ;
#30179=DIRECTION ( 'NONE',  ( -0.000000000000000000, 0.000000000000000000, -1.000000000000000000 ) ) ;
#30206=CARTESIAN_POINT ( 'NONE',  ( 3.999999999999997335, 7.500000000000000888, 14.00000000000000178 ) ) ;
#30359=VERTEX_POINT ( 'NONE', #3184 ) ;
#30415=CYLINDRICAL_SURFACE ( 'NONE', #70560, 1.999999999999998224 ) ;
#30436=ORIENTED_EDGE ( 'NONE', *, *, #9324, .F. ) ;
#30457=EDGE_LOOP ( 'NONE', ( #45895, #88124, #77143, #79630 ) ) ;
#30465=DIRECTION ( 'NONE',  ( -1.000000000000000000, 0.000000000000000000, 0.000000000000000000 ) ) ;
#30483=DIRECTION ( 'NONE',  ( -0.000000000000000000, 0.000000000000000000, -1.000000000000000000 ) ) ;
#30487=DIRECTION ( 'NONE',  ( 0.000000000000000000, 0.000000000000000000, 1.000000000000000000 ) ) ;
#30553=ORIENTED_EDGE ( 'NONE', *, *, #70435, .F. ) ;
#30623=EDGE_CURVE ( 'NONE', #62427, #4695, #25102, .T. ) ;
#30695=DIRECTION ( 'NONE',  ( 0.000000000000000000, 0.000000000000000000, 1.000000000000000000 ) ) ;
#30801=DIRECTION ( 'NONE',  ( 1.000000000000000000, 0.000000000000000000, 0.000000000000000000 ) ) ;
#30833=DIRECTION ( 'NONE',  ( -0.000000000000000000, -0.000000000000000000, -1.000000000000000000 ) ) ;
#30888=CARTESIAN_POINT ( 'NONE',  ( 19.99999999999996803, 15.00000000000000711, 3.000000000000000000 ) ) ;
#30956=LINE ( 'NONE', #51660, #24462 ) ;
#31119=CARTESIAN_POINT ( 'NONE',  ( -19.99999999999998934, 12.00000000000000711, 10.00000000000000178 ) ) ;
#31251=AXIS2_PLACEMENT_3D ( 'NONE', #28043, #8672, #61822 ) ;
#31293=VERTEX_POINT ( 'NONE', #22694 ) ;
#31320=VERTEX_POINT ( 'NONE', #78085 ) ;
#31399=CARTESIAN_POINT ( 'NONE',  ( 1.653273178848927064E-15, -7.500000000000000000, 13.50000000000000178 ) ) ;
#31413=APPLICATION_CONTEXT ( 'automotive_design' ) ;
#31447=ORIENTED_EDGE ( 'NONE', *, *, #58155, .T. ) ;
#31499=VERTEX_POINT ( 'NONE', #87087 ) ;
#31525=DIRECTION ( 'NONE',  ( 2.891205793294679312E-16, -1.000000000000000000, 0.000000000000000000 ) ) ;
#31535=ORIENTED_EDGE ( 'NONE', *, *, #54468, .F. ) ;
#31557=LINE ( 'NONE', #86520, #39302 ) ;
#31662=LINE ( 'NONE', #18149, #40864 ) ;
#31714=DIRECTION ( 'NONE',  ( 0.000000000000000000, 0.000000000000000000, 1.000000000000000000 ) ) ;
#31715=ORIENTED_EDGE ( 'NONE', *, *, #79931, .T. ) ;
#31734=DIRECTION ( 'NONE',  ( 0.000000000000000000, 0.000000000000000000, 1.000000000000000000 ) ) ;
#31767=DIRECTION ( 'NONE',  ( -0.000000000000000000, -0.000000000000000000, -1.000000000000000000 ) ) ;
#31785=DIRECTION ( 'NONE',  ( 0.000000000000000000, 1.000000000000000000, 0.000000000000000000 ) ) ;
#31813=CARTESIAN_POINT ( 'NONE',  ( 20.00000000000000355, 10.00000000000000533, 13.00000000000000178 ) ) ;
#31862=PLANE ( 'NONE',  #35337 ) ;
#31863=ADVANCED_FACE ( 'NONE', ( #89087, #68787 ), #75538, .T. ) ;
#31891=ORIENTED_EDGE ( 'NONE', *, *, #66233, .F. ) ;
#31913=CARTESIAN_POINT ( 'NONE',  ( 24.99999999999999645, -15.00000000000000000, 3.000000000000000000 ) ) ;
#31918=CARTESIAN_POINT ( 'NONE',  ( 3.000000000000001776, -7.500000000000000000, 14.00000000000000178 ) ) ;
#31919=EDGE_LOOP ( 'NONE', ( #42853, #61389, #2200, #35798 ) ) ;
#31988=PRODUCT ( 'head base', 'head base', '', ( #5915 ) ) ;
#32033=ORIENTED_EDGE ( 'NONE', *, *, #34301, .T. ) ;
#32052=SHAPE_DEFINITION_REPRESENTATION ( #57813, #85713 ) ;
#32077=DIRECTION ( 'NONE',  ( 1.000000000000000000, 0.000000000000000000, 0.000000000000000000 ) ) ;
#32114=CIRCLE ( 'NONE', #20594, 4.000000000000000000 ) ;
#32170=VERTEX_POINT ( 'NONE', #30888 ) ;
#32182=CARTESIAN_POINT ( 'NONE',  ( -20.00000000000000355, 10.00000000000000711, 3.000000000000000000 ) ) ;
#32213=VERTEX_POINT ( 'NONE', #52048 ) ;
#32228=DIRECTION ( 'NONE',  ( 0.000000000000000000, -0.000000000000000000, 1.000000000000000000 ) ) ;
#32256=DIRECTION ( 'NONE',  ( -1.000000000000000000, 0.000000000000000000, 0.000000000000000000 ) ) ;
#32287=ADVANCED_FACE ( 'NONE', ( #83090, #20928, #19606 ), #75005, .T. ) ;
#32432=VECTOR ( 'NONE', #30833, 1000.000000000000000 ) ;
#32507=EDGE_CURVE ( 'NONE', #33215, #63487, #68185, .T. ) ;
#32554=VECTOR ( 'NONE', #18919, 1000.000000000000000 ) ;
#32864=DIRECTION ( 'NONE',  ( -1.000000000000000000, 0.000000000000000000, 0.000000000000000000 ) ) ;
#32910=VECTOR ( 'NONE', #82235, 1000.000000000000000 ) ;
#32938=FACE_OUTER_BOUND ( 'NONE', #77732, .T. ) ;
#33010=ADVANCED_FACE ( 'NONE', ( #42549 ), #21827, .T. ) ;
#33116=ORIENTED_EDGE ( 'NONE', *, *, #60734, .T. ) ;
#33181=CARTESIAN_POINT ( 'NONE',  ( 30.00000000000000000, -15.00000000000000000, 3.000000000000000000 ) ) ;
#33215=VERTEX_POINT ( 'NONE', #51042 ) ;
#33352=PLANE ( 'NONE',  #78963 ) ;
#33378=AXIS2_PLACEMENT_3D ( 'NONE', #67175, #27514, #73937 ) ;
#33385=DIRECTION ( 'NONE',  ( -1.734723475976812518E-16, 1.000000000000000000, 0.000000000000000000 ) ) ;
#33418=ORIENTED_EDGE ( 'NONE', *, *, #34261, .T. ) ;
#33484=DIRECTION ( 'NONE',  ( 1.000000000000000000, 2.602085213965214586E-16, 0.000000000000000000 ) ) ;
#33584=VERTEX_POINT ( 'NONE', #40136 ) ;
#33657=CARTESIAN_POINT ( 'NONE',  ( 19.99999999999996803, 15.00000000000000711, 13.00000000000000178 ) ) ;
#33666=DIRECTION ( 'NONE',  ( -0.000000000000000000, -0.000000000000000000, -1.000000000000000000 ) ) ;
#33896=ADVANCED_FACE ( 'NONE', ( #79225, #17524 ), #18855, .T. ) ;
#33956=FACE_OUTER_BOUND ( 'NONE', #25593, .T. ) ;
#33997=ORIENTED_EDGE ( 'NONE', *, *, #7623, .T. ) ;
#34010=VERTEX_POINT ( 'NONE', #12545 ) ;
#34045=CARTESIAN_POINT ( 'NONE',  ( -4.500000000000003553, 7.499999999999996447, 13.50000000000000178 ) ) ;
#34053=VERTEX_POINT ( 'NONE', #1234 ) ;
#34092=LINE ( 'NONE', #33657, #16805 ) ;
#34095=ORIENTED_EDGE ( 'NONE', *, *, #65557, .T. ) ;
#34162=CARTESIAN_POINT ( 'NONE',  ( -25.00000000000000000, -10.00000000000000533, 13.00000000000000178 ) ) ;
#34261=EDGE_CURVE ( 'NONE', #60372, #22195, #45272, .T. ) ;
#34301=EDGE_CURVE ( 'NONE', #22580, #14205, #76916, .T. ) ;
#34378=CARTESIAN_POINT ( 'NONE',  ( -22.00000000000000355, -15.00000000000000000, 0.000000000000000000 ) ) ;
#34399=DIRECTION ( 'NONE',  ( -0.000000000000000000, -0.000000000000000000, -1.000000000000000000 ) ) ;
#34540=ORIENTED_EDGE ( 'NONE', *, *, #81297, .T. ) ;
#34844=DIRECTION ( 'NONE',  ( -0.000000000000000000, -1.000000000000000000, -0.000000000000000000 ) ) ;
#34986=CARTESIAN_POINT ( 'NONE',  ( -19.99999999999996447, -12.00000000000000355, 10.00000000000000178 ) ) ;
#34993=ORIENTED_EDGE ( 'NONE', *, *, #36655, .T. ) ;
#35070=CIRCLE ( 'NONE', #73979, 3.000000000000000000 ) ;
#35236=ORIENTED_EDGE ( 'NONE', *, *, #40107, .T. ) ;
#35307=DIRECTION ( 'NONE',  ( 1.000000000000000000, 0.000000000000000000, 0.000000000000000000 ) ) ;
#35337=AXIS2_PLACEMENT_3D ( 'NONE', #45805, #60649, #60206 ) ;
#35366=LINE ( 'NONE', #61944, #32910 ) ;
#35389=CARTESIAN_POINT ( 'NONE',  ( 4.500000000000003553, -7.499999999999998224, 13.00000000000000178 ) ) ;
#35442=DIRECTION ( 'NONE',  ( 1.000000000000000000, 0.000000000000000000, -0.000000000000000000 ) ) ;
#35447=CIRCLE ( 'NONE', #57602, 3.000000000000000000 ) ;
#35454=ORIENTED_EDGE ( 'NONE', *, *, #64434, .T. ) ;
#35525=CYLINDRICAL_SURFACE ( 'NONE', #54308, 4.500000000000001776 ) ;
#35603=EDGE_CURVE ( 'NONE', #59616, #82973, #16438, .T. ) ;
#35683=ORIENTED_EDGE ( 'NONE', *, *, #35603, .F. ) ;
#35765=FILL_AREA_STYLE ('',( #70876 ) ) ;
#35779=CARTESIAN_POINT ( 'NONE',  ( 25.00000000000000355, 9.999999999999971578, 13.00000000000000178 ) ) ;
#35788=EDGE_LOOP ( 'NONE', ( #71125, #59406, #21708, #25187 ) ) ;
#35798=ORIENTED_EDGE ( 'NONE', *, *, #54468, .T. ) ;
#35857=CARTESIAN_POINT ( 'NONE',  ( 1.653273178848927064E-15, -7.500000000000000000, 13.50000000000000178 ) ) ;
#35872=VECTOR ( 'NONE', #2378, 1000.000000000000000 ) ;
#35902=LINE ( 'NONE', #2534, #22863 ) ;
#35970=DIRECTION ( 'NONE',  ( 1.000000000000000000, 0.000000000000000000, 0.000000000000000000 ) ) ;
#36090=ORIENTED_EDGE ( 'NONE', *, *, #41283, .T. ) ;
#36136=EDGE_CURVE ( 'NONE', #31320, #15649, #13768, .T. ) ;
#36183=EDGE_CURVE ( 'NONE', #82502, #68350, #39927, .T. ) ;
#36308=DIRECTION ( 'NONE',  ( -1.000000000000000000, 5.637851296924618008E-14, 0.000000000000000000 ) ) ;
#36433=DIRECTION ( 'NONE',  ( 1.000000000000000000, 0.000000000000000000, 0.000000000000000000 ) ) ;
#36443=CARTESIAN_POINT ( 'NONE',  ( -24.99999999999999645, 20.00000000000000355, 3.000000000000000000 ) ) ;
#36655=EDGE_CURVE ( 'NONE', #71705, #67458, #27629, .T. ) ;
#36784=ORIENTED_EDGE ( 'NONE', *, *, #27715, .F. ) ;
#36794=CARTESIAN_POINT ( 'NONE',  ( -19.99999999999996447, -12.00000000000000355, 13.00000000000000178 ) ) ;
#36806=CARTESIAN_POINT ( 'NONE',  ( -20.00000000000000355, -10.00000000000000533, 0.000000000000000000 ) ) ;
#36820=CARTESIAN_POINT ( 'NONE',  ( -2.939152317953646711E-15, 7.500000000000000000, 14.00000000000000178 ) ) ;
#36862=AXIS2_PLACEMENT_3D ( 'NONE', #1409, #29774, #8623 ) ;
#36898=VERTEX_POINT ( 'NONE', #18115 ) ;
#36917=CYLINDRICAL_SURFACE ( 'NONE', #42070, 5.000000000000000888 ) ;
#37043=VERTEX_POINT ( 'NONE', #60867 ) ;
#37077=ADVANCED_FACE ( 'NONE', ( #87475 ), #41485, .F. ) ;
#37163=FACE_OUTER_BOUND ( 'NONE', #17093, .T. ) ;
#37350=AXIS2_PLACEMENT_3D ( 'NONE', #84255, #30179, #57647 ) ;
#37576=EDGE_LOOP ( 'NONE', ( #23923, #15638, #53734, #57793 ) ) ;
#37931=CIRCLE ( 'NONE', #55222, 4.000000000000000000 ) ;
#37933=FACE_OUTER_BOUND ( 'NONE', #19175, .T. ) ;
#37946=DIRECTION ( 'NONE',  ( 0.000000000000000000, 0.000000000000000000, 1.000000000000000000 ) ) ;
#37978=ORIENTED_EDGE ( 'NONE', *, *, #84164, .T. ) ;
#38114=VERTEX_POINT ( 'NONE', #30206 ) ;
#38130=SURFACE_STYLE_FILL_AREA ( #10663 ) ;
#38200=VERTEX_POINT ( 'NONE', #14361 ) ;
#38247=CARTESIAN_POINT ( 'NONE',  ( -22.00000000000000711, 9.999999999999971578, 13.00000000000000178 ) ) ;
#38282=EDGE_CURVE ( 'NONE', #73496, #10700, #25474, .T. ) ;
#38441=CIRCLE ( 'NONE', #68591, 4.500000000000001776 ) ;
#38465=VERTEX_POINT ( 'NONE', #64094 ) ;
#38501=CIRCLE ( 'NONE', #86003, 3.000000000000000444 ) ;
#38505=ORIENTED_EDGE ( 'NONE', *, *, #53106, .T. ) ;
#38627=CARTESIAN_POINT ( 'NONE',  ( -2.939152317953646711E-15, 7.500000000000000000, 10.00000000000000178 ) ) ;
#38639=EDGE_LOOP ( 'NONE', ( #77939, #31535, #73452, #33116 ) ) ;
#38761=AXIS2_PLACEMENT_3D ( 'NONE', #71324, #29916, #4204 ) ;
#38842=DIRECTION ( 'NONE',  ( 2.891205793294678326E-16, -1.000000000000000000, 0.000000000000000000 ) ) ;
#38846=CARTESIAN_POINT ( 'NONE',  ( 1.653273178848927064E-15, -7.500000000000000000, 14.00000000000000178 ) ) ;
#38887=CIRCLE ( 'NONE', #73416, 5.000000000000000888 ) ;
#38920=DIRECTION ( 'NONE',  ( -0.000000000000000000, -0.000000000000000000, -1.000000000000000000 ) ) ;
#39157=CARTESIAN_POINT ( 'NONE',  ( -25.00000000000000000, -10.00000000000000533, 3.000000000000000000 ) ) ;
#39224=EDGE_CURVE ( 'NONE', #17051, #81438, #72988, .T. ) ;
#39302=VECTOR ( 'NONE', #24795, 1000.000000000000000 ) ;
#39465=DIRECTION ( 'NONE',  ( 0.000000000000000000, 0.000000000000000000, 1.000000000000000000 ) ) ;
#39480=DIRECTION ( 'NONE',  ( 1.000000000000000000, 0.000000000000000000, 0.000000000000000000 ) ) ;
#39605=DIRECTION ( 'NONE',  ( -1.000000000000000000, -0.000000000000000000, -0.000000000000000000 ) ) ;
#39637=CARTESIAN_POINT ( 'NONE',  ( 20.00000000000000355, 10.00000000000000533, 3.000000000000000000 ) ) ;
#39671=DIRECTION ( 'NONE',  ( -0.000000000000000000, -0.000000000000000000, -1.000000000000000000 ) ) ;
#39749=DIRECTION ( 'NONE',  ( 1.000000000000000000, 0.000000000000000000, 0.000000000000000000 ) ) ;
#39784=DIRECTION ( 'NONE',  ( -0.000000000000000000, -0.000000000000000000, -1.000000000000000000 ) ) ;
#39921=DIRECTION ( 'NONE',  ( 0.000000000000000000, -1.000000000000000000, 0.000000000000000000 ) ) ;
#39927=LINE ( 'NONE', #58388, #5172 ) ;
#39955=DIRECTION ( 'NONE',  ( 1.000000000000000000, 0.000000000000000000, 0.000000000000000000 ) ) ;
#39980=DIRECTION ( 'NONE',  ( 0.000000000000000000, 0.000000000000000000, 1.000000000000000000 ) ) ;
#40055=ORIENTED_EDGE ( 'NONE', *, *, #62373, .T. ) ;
#40107=EDGE_CURVE ( 'NONE', #63332, #68729, #80812, .T. ) ;
#40136=CARTESIAN_POINT ( 'NONE',  ( -30.00000000000000000, -15.00000000000000000, 3.000000000000000000 ) ) ;
#40151=DIRECTION ( 'NONE',  ( 1.000000000000000000, 1.734723475976812518E-16, -0.000000000000000000 ) ) ;
#40270=VERTEX_POINT ( 'NONE', #17662 ) ;
#40287=ORIENTED_EDGE ( 'NONE', *, *, #1802, .F. ) ;
#40303=AXIS2_PLACEMENT_3D ( 'NONE', #32182, #46137, #73628 ) ;
#40396=LINE ( 'NONE', #33181, #76287 ) ;
#40427=EDGE_LOOP ( 'NONE', ( #75654, #42220, #47719, #35683 ) ) ;
#40435=CYLINDRICAL_SURFACE ( 'NONE', #87518, 2.000000000000001776 ) ;
#40436=CARTESIAN_POINT ( 'NONE',  ( 1.653273178848927064E-15, -7.500000000000000000, 14.00000000000000178 ) ) ;
#40438=CIRCLE ( 'NONE', #27496, 3.000000000000000444 ) ;
#40720=CARTESIAN_POINT ( 'NONE',  ( 19.99999999999999289, -11.99999999999999467, 13.00000000000000178 ) ) ;
#40864=VECTOR ( 'NONE', #19474, 1000.000000000000000 ) ;
#40868=DIRECTION ( 'NONE',  ( -1.000000000000000000, 0.000000000000000000, 0.000000000000000000 ) ) ;
#40908=DIRECTION ( 'NONE',  ( 0.000000000000000000, -0.000000000000000000, -1.000000000000000000 ) ) ;
#40973=EDGE_CURVE ( 'NONE', #14205, #31293, #78244, .T. ) ;
#40982=AXIS2_PLACEMENT_3D ( 'NONE', #41128, #20413, #46980 ) ;
#41128=CARTESIAN_POINT ( 'NONE',  ( -20.00000000000000355, -10.00000000000000533, 3.000000000000000000 ) ) ;
#41283=EDGE_CURVE ( 'NONE', #19865, #59616, #87703, .T. ) ;
#41485=PLANE ( 'NONE',  #46882 ) ;
#41495=ORIENTED_EDGE ( 'NONE', *, *, #30623, .T. ) ;
#41583=EDGE_LOOP ( 'NONE', ( #10429, #78790, #74270, #73429 ) ) ;
#41723=EDGE_CURVE ( 'NONE', #17051, #22580, #6281, .T. ) ;
#41745=ORIENTED_EDGE ( 'NONE', *, *, #55433, .T. ) ;
#41847=CARTESIAN_POINT ( 'NONE',  ( 22.00000000000000711, 9.999999999999991118, 13.00000000000000178 ) ) ;
#41992=ORIENTED_EDGE ( 'NONE', *, *, #47035, .F. ) ;
#41994=CYLINDRICAL_SURFACE ( 'NONE', #64894, 3.000000000000000444 ) ;
#42003=EDGE_CURVE ( 'NONE', #2192, #82502, #30956, .T. ) ;
#42070=AXIS2_PLACEMENT_3D ( 'NONE', #47229, #81482, #67071 ) ;
#42081=( NAMED_UNIT ( * ) PLANE_ANGLE_UNIT ( ) SI_UNIT ( $, .RADIAN. ) );
#42082=PLANE ( 'NONE',  #59910 ) ;
#42220=ORIENTED_EDGE ( 'NONE', *, *, #2087, .T. ) ;
#42311=ORIENTED_EDGE ( 'NONE', *, *, #68582, .T. ) ;
#42547=AXIS2_PLACEMENT_3D ( 'NONE', #38846, #78481, #17229 ) ;
#42549=FACE_OUTER_BOUND ( 'NONE', #73172, .T. ) ;
#42626=EDGE_CURVE ( 'NONE', #34010, #8684, #12470, .T. ) ;
#42643=DIRECTION ( 'NONE',  ( 1.000000000000000000, 2.602085213965214586E-16, -0.000000000000000000 ) ) ;
#42648=PLANE ( 'NONE',  #21386 ) ;
#42675=CARTESIAN_POINT ( 'NONE',  ( 19.99999999999997158, -14.99999999999999467, 13.00000000000000178 ) ) ;
#42732=ORIENTED_EDGE ( 'NONE', *, *, #28372, .T. ) ;
#42774=CYLINDRICAL_SURFACE ( 'NONE', #61758, 5.000000000000000888 ) ;
#42777=ADVANCED_FACE ( 'NONE', ( #79045 ), #57434, .F. ) ;
#42792=EDGE_CURVE ( 'NONE', #38465, #53590, #38887, .T. ) ;
#42819=PLANE ( 'NONE',  #37350 ) ;
#42853=ORIENTED_EDGE ( 'NONE', *, *, #32507, .T. ) ;
#42961=SURFACE_STYLE_USAGE ( .BOTH. , #63214 ) ;
#42983=DIRECTION ( 'NONE',  ( 0.000000000000000000, 0.000000000000000000, 1.000000000000000000 ) ) ;
#43137=CARTESIAN_POINT ( 'NONE',  ( -19.99999999999996803, 15.00000000000000711, 13.00000000000000178 ) ) ;
#43326=DIRECTION ( 'NONE',  ( 1.000000000000000000, 0.000000000000000000, -0.000000000000000000 ) ) ;
#43345=ADVANCED_FACE ( 'NONE', ( #55343 ), #35525, .T. ) ;
#43347=ORIENTED_EDGE ( 'NONE', *, *, #76416, .F. ) ;
#43412=AXIS2_PLACEMENT_3D ( 'NONE', #45596, #73074, #39749 ) ;
#43568=DIRECTION ( 'NONE',  ( -0.000000000000000000, -0.000000000000000000, -1.000000000000000000 ) ) ;
#43713=UNCERTAINTY_MEASURE_WITH_UNIT (LENGTH_MEASURE( 1.000000000000000082E-05 ), #56899, 'distance_accuracy_value', 'NONE');
#43730=CARTESIAN_POINT ( 'NONE',  ( -19.99999999999998934, 12.00000000000000711, 13.00000000000000178 ) ) ;
#43741=CIRCLE ( 'NONE', #4928, 5.000000000000000888 ) ;
#43792=EDGE_LOOP ( 'NONE', ( #83158, #78850, #10890, #20587 ) ) ;
#43871=ADVANCED_FACE ( 'NONE', ( #79058 ), #43937, .T. ) ;
#43880=LINE ( 'NONE', #59617, #64379 ) ;
#43907=CARTESIAN_POINT ( 'NONE',  ( -3.999999999999998224, -7.500000000000000000, 14.00000000000000178 ) ) ;
#43922=CARTESIAN_POINT ( 'NONE',  ( 24.99999999999999645, 20.00000000000000355, 3.000000000000000000 ) ) ;
#43937=CYLINDRICAL_SURFACE ( 'NONE', #15556, 4.500000000000001776 ) ;
#44101=CARTESIAN_POINT ( 'NONE',  ( -20.00000000000000355, 10.00000000000000711, 10.00000000000000178 ) ) ;
#44218=CARTESIAN_POINT ( 'NONE',  ( 24.99999999999999645, 15.00000000000000355, 3.000000000000000000 ) ) ;
#44356=EDGE_CURVE ( 'NONE', #25459, #82973, #29898, .T. ) ;
#44377=VECTOR ( 'NONE', #78593, 1000.000000000000000 ) ;
#44443=FACE_OUTER_BOUND ( 'NONE', #60089, .T. ) ;
#44444=CARTESIAN_POINT ( 'NONE',  ( -19.99999999999996447, -15.00000000000000533, 3.000000000000000000 ) ) ;
#44473=DIRECTION ( 'NONE',  ( 0.000000000000000000, 0.000000000000000000, 1.000000000000000000 ) ) ;
#44509=DIRECTION ( 'NONE',  ( 1.000000000000000000, 0.000000000000000000, 0.000000000000000000 ) ) ;
#44629=CARTESIAN_POINT ( 'NONE',  ( -24.99999999999999645, 20.00000000000000355, 3.000000000000000000 ) ) ;
#44780=CARTESIAN_POINT ( 'NONE',  ( 24.99999999999999645, -15.00000000000000000, 0.000000000000000000 ) ) ;
#44802=DIRECTION ( 'NONE',  ( -0.000000000000000000, -0.000000000000000000, -1.000000000000000000 ) ) ;
#44852=EDGE_LOOP ( 'NONE', ( #36784, #64801 ) ) ;
#44929=ORIENTED_EDGE ( 'NONE', *, *, #1205, .F. ) ;
#45272=CIRCLE ( 'NONE', #69709, 1.999999999999998224 ) ;
#45329=DIRECTION ( 'NONE',  ( -1.000000000000000000, -0.000000000000000000, -0.000000000000000000 ) ) ;
#45421=AXIS2_PLACEMENT_3D ( 'NONE', #57100, #71058, #85911 ) ;
#45437=DIRECTION ( 'NONE',  ( -0.000000000000000000, -0.000000000000000000, -1.000000000000000000 ) ) ;
#45596=CARTESIAN_POINT ( 'NONE',  ( 20.00000000000000711, -9.999999999999994671, 10.00000000000000178 ) ) ;
#45704=VECTOR ( 'NONE', #52105, 1000.000000000000000 ) ;
#45737=ORIENTED_EDGE ( 'NONE', *, *, #67363, .T. ) ;
#45805=CARTESIAN_POINT ( 'NONE',  ( -19.99999999999996447, -12.00000000000000355, 13.00000000000000178 ) ) ;
#45895=ORIENTED_EDGE ( 'NONE', *, *, #23274, .T. ) ;
#45956=CYLINDRICAL_SURFACE ( 'NONE', #30007, 4.000000000000000000 ) ;
#46019=ORIENTED_EDGE ( 'NONE', *, *, #29865, .F. ) ;
#46084=ORIENTED_EDGE ( 'NONE', *, *, #46164, .T. ) ;
#46134=DIRECTION ( 'NONE',  ( 1.000000000000000000, 0.000000000000000000, 0.000000000000000000 ) ) ;
#46137=DIRECTION ( 'NONE',  ( 0.000000000000000000, 0.000000000000000000, 1.000000000000000000 ) ) ;
#46147=AXIS2_PLACEMENT_3D ( 'NONE', #15476, #8719, #16783 ) ;
#46155=ADVANCED_FACE ( 'NONE', ( #86795 ), #25066, .F. ) ;
#46164=EDGE_CURVE ( 'NONE', #3413, #55616, #35366, .T. ) ;
#46348=EDGE_LOOP ( 'NONE', ( #62884, #54169, #24724, #3039 ) ) ;
#46367=LINE ( 'NONE', #24761, #28373 ) ;
#46464=DIRECTION ( 'NONE',  ( 1.000000000000000000, 0.000000000000000000, 0.000000000000000000 ) ) ;
#46490=CIRCLE ( 'NONE', #11970, 4.000000000000000000 ) ;
#46610=ORIENTED_EDGE ( 'NONE', *, *, #68582, .F. ) ;
#46619=ORIENTED_EDGE ( 'NONE', *, *, #73665, .T. ) ;
#46787=CARTESIAN_POINT ( 'NONE',  ( -24.99999999999999645, 20.00000000000000355, 0.000000000000000000 ) ) ;
#46854=CARTESIAN_POINT ( 'NONE',  ( 22.00000000000000711, 9.999999999999971578, 13.00000000000000178 ) ) ;
#46882=AXIS2_PLACEMENT_3D ( 'NONE', #13129, #61739, #25755 ) ;
#46900=ORIENTED_EDGE ( 'NONE', *, *, #79931, .F. ) ;
#46934=DIRECTION ( 'NONE',  ( 1.000000000000000000, 0.000000000000000000, 0.000000000000000000 ) ) ;
#46958=EDGE_CURVE ( 'NONE', #82973, #25459, #71594, .T. ) ;
#46980=DIRECTION ( 'NONE',  ( -1.000000000000000000, 0.000000000000000000, 0.000000000000000000 ) ) ;
#46985=DIRECTION ( 'NONE',  ( -0.000000000000000000, -0.000000000000000000, -1.000000000000000000 ) ) ;
#46988=ORIENTED_EDGE ( 'NONE', *, *, #32507, .F. ) ;
#47035=EDGE_CURVE ( 'NONE', #31499, #85628, #9794, .T. ) ;
#47091=EDGE_LOOP ( 'NONE', ( #46619, #7983, #49455, #1060 ) ) ;
#47183=EDGE_LOOP ( 'NONE', ( #19558, #38505 ) ) ;
#47229=CARTESIAN_POINT ( 'NONE',  ( -20.00000000000000355, 10.00000000000000711, 13.00000000000000178 ) ) ;
#47363=CIRCLE ( 'NONE', #87635, 5.000000000000000888 ) ;
#47464=ORIENTED_EDGE ( 'NONE', *, *, #49867, .F. ) ;
#47553=DIRECTION ( 'NONE',  ( -2.891205793294679312E-16, 1.000000000000000000, 0.000000000000000000 ) ) ;
#47700=ADVANCED_FACE ( 'NONE', ( #12944 ), #40435, .F. ) ;
#47719=ORIENTED_EDGE ( 'NONE', *, *, #44356, .T. ) ;
#47720=CIRCLE ( 'NONE', #43412, 1.999999999999998224 ) ;
#48025=DIRECTION ( 'NONE',  ( 0.000000000000000000, 0.000000000000000000, 1.000000000000000000 ) ) ;
#48049=DIRECTION ( 'NONE',  ( 0.000000000000000000, 0.000000000000000000, 1.000000000000000000 ) ) ;
#48307=ADVANCED_FACE ( 'NONE', ( #86526 ), #45956, .T. ) ;
#48601=ADVANCED_FACE ( 'NONE', ( #80540 ), #65222, .F. ) ;
#48737=VECTOR ( 'NONE', #68181, 1000.000000000000000 ) ;
#48810=VECTOR ( 'NONE', #6906, 1000.000000000000000 ) ;
#48813=ADVANCED_FACE ( 'NONE', ( #62452 ), #42648, .F. ) ;
#48930=LINE ( 'NONE', #76403, #57898 ) ;
#48941=CARTESIAN_POINT ( 'NONE',  ( 19.99999999999996803, 15.00000000000000711, 13.00000000000000178 ) ) ;
#48965=ORIENTED_EDGE ( 'NONE', *, *, #19711, .F. ) ;
#49192=EDGE_LOOP ( 'NONE', ( #1177, #21371, #35454, #62564 ) ) ;
#49270=( LENGTH_UNIT ( ) NAMED_UNIT ( * ) SI_UNIT ( .MILLI., .METRE. ) );
#49276=ADVANCED_FACE ( 'NONE', ( #51476 ), #16389, .F. ) ;
#49344=CARTESIAN_POINT ( 'NONE',  ( 25.00000000000000711, -9.999999999999957367, 13.00000000000000178 ) ) ;
#49391=LINE ( 'NONE', #6632, #76642 ) ;
#49437=ADVANCED_FACE ( 'NONE', ( #1770 ), #29696, .T. ) ;
#49455=ORIENTED_EDGE ( 'NONE', *, *, #75759, .F. ) ;
#49482=ORIENTED_EDGE ( 'NONE', *, *, #27409, .F. ) ;
#49596=EDGE_CURVE ( 'NONE', #55616, #18826, #47363, .T. ) ;
#49672=ORIENTED_EDGE ( 'NONE', *, *, #40973, .F. ) ;
#49808=CARTESIAN_POINT ( 'NONE',  ( 24.99999999999999645, -15.00000000000000000, 3.000000000000000000 ) ) ;
#49853=EDGE_CURVE ( 'NONE', #79858, #82502, #4219, .T. ) ;
#49867=EDGE_CURVE ( 'NONE', #55616, #8684, #35902, .T. ) ;
#50100=ORIENTED_EDGE ( 'NONE', *, *, #18066, .T. ) ;
#50125=AXIS2_PLACEMENT_3D ( 'NONE', #87304, #72424, #25134 ) ;
#50161=CARTESIAN_POINT ( 'NONE',  ( -2.999999999999998224, -7.500000000000000000, 0.000000000000000000 ) ) ;
#50204=CARTESIAN_POINT ( 'NONE',  ( -19.99999999999996803, 12.00000000000000711, 10.00000000000000178 ) ) ;
#50215=EDGE_LOOP ( 'NONE', ( #26789, #66223, #24007, #72370 ) ) ;
#50276=CARTESIAN_POINT ( 'NONE',  ( -20.00000000000000355, -10.00000000000000533, 13.00000000000000178 ) ) ;
#50332=FACE_OUTER_BOUND ( 'NONE', #47091, .T. ) ;
#50469=ORIENTED_EDGE ( 'NONE', *, *, #64186, .F. ) ;
#50681=ADVANCED_FACE ( 'NONE', ( #13959 ), #42774, .T. ) ;
#50943=VERTEX_POINT ( 'NONE', #80998 ) ;
#50991=DIRECTION ( 'NONE',  ( -1.734723475976813750E-16, 1.000000000000000000, -0.000000000000000000 ) ) ;
#51011=VERTEX_POINT ( 'NONE', #82326 ) ;
#51042=CARTESIAN_POINT ( 'NONE',  ( -4.500000000000000000, -7.499999999999999112, 13.00000000000000178 ) ) ;
#51163=CARTESIAN_POINT ( 'NONE',  ( 20.00000000000000711, -9.999999999999994671, 0.000000000000000000 ) ) ;
#51203=LINE ( 'NONE', #64291, #72103 ) ;
#51280=EDGE_CURVE ( 'NONE', #2315, #18545, #83442, .T. ) ;
#51310=DIRECTION ( 'NONE',  ( -1.000000000000000000, 0.000000000000000000, 0.000000000000000000 ) ) ;
#51337=ORIENTED_EDGE ( 'NONE', *, *, #54583, .F. ) ;
#51417=ORIENTED_EDGE ( 'NONE', *, *, #49853, .F. ) ;
#51476=FACE_OUTER_BOUND ( 'NONE', #15394, .T. ) ;
#51660=CARTESIAN_POINT ( 'NONE',  ( 19.99999999999996803, 12.00000000000000711, 13.00000000000000178 ) ) ;
#51880=DIRECTION ( 'NONE',  ( -1.000000000000000000, -2.891205793294678326E-16, 0.000000000000000000 ) ) ;
#51960=DIRECTION ( 'NONE',  ( 1.000000000000000000, 0.000000000000000000, 0.000000000000000000 ) ) ;
#52048=CARTESIAN_POINT ( 'NONE',  ( -19.99999999999996447, -12.00000000000000355, 0.000000000000000000 ) ) ;
#52080=ORIENTED_EDGE ( 'NONE', *, *, #51280, .T. ) ;
#52099=ORIENTED_EDGE ( 'NONE', *, *, #6846, .F. ) ;
#52105=DIRECTION ( 'NONE',  ( -2.891205793294678326E-16, 1.000000000000000000, -0.000000000000000000 ) ) ;
#52247=CARTESIAN_POINT ( 'NONE',  ( 4.499999999999999112, 7.500000000000002665, 13.00000000000000178 ) ) ;
#52351=EDGE_LOOP ( 'NONE', ( #44929, #195, #42311, #14937 ) ) ;
#52526=ORIENTED_EDGE ( 'NONE', *, *, #54583, .T. ) ;
#52527=CARTESIAN_POINT ( 'NONE',  ( 1.653273178848927064E-15, -7.500000000000000000, 0.000000000000000000 ) ) ;
#52646=DIRECTION ( 'NONE',  ( 2.891205793294679312E-16, -1.000000000000000000, 0.000000000000000000 ) ) ;
#52692=LINE ( 'NONE', #52247, #32554 ) ;
#52732=CARTESIAN_POINT ( 'NONE',  ( 4.000000000000001776, -7.499999999999999112, 13.50000000000000178 ) ) ;
#52842=EDGE_LOOP ( 'NONE', ( #73431, #87752, #10748, #83551 ) ) ;
#53020=DIRECTION ( 'NONE',  ( -0.000000000000000000, -0.000000000000000000, 1.000000000000000000 ) ) ;
#53106=EDGE_CURVE ( 'NONE', #10700, #73496, #40438, .T. ) ;
#53111=CIRCLE ( 'NONE', #83290, 5.000000000000000888 ) ;
#53210=AXIS2_PLACEMENT_3D ( 'NONE', #17223, #66299, #65843 ) ;
#53249=PLANE ( 'NONE',  #26046 ) ;
#53279=EDGE_CURVE ( 'NONE', #62427, #79550, #15667, .T. ) ;
#53403=CARTESIAN_POINT ( 'NONE',  ( -4.000000000000002665, 7.500000000000000000, 14.00000000000000178 ) ) ;
#53590=VERTEX_POINT ( 'NONE', #49344 ) ;
#53699=ADVANCED_FACE ( 'NONE', ( #7760 ), #41994, .F. ) ;
#53734=ORIENTED_EDGE ( 'NONE', *, *, #7623, .F. ) ;
#53774=DIRECTION ( 'NONE',  ( 0.000000000000000000, 0.000000000000000000, 1.000000000000000000 ) ) ;
#53834=DIRECTION ( 'NONE',  ( 0.000000000000000000, 0.000000000000000000, 1.000000000000000000 ) ) ;
#53982=LINE ( 'NONE', #19757, #66238 ) ;
#54043=VECTOR ( 'NONE', #50991, 1000.000000000000000 ) ;
#54169=ORIENTED_EDGE ( 'NONE', *, *, #30110, .F. ) ;
#54212=EDGE_CURVE ( 'NONE', #22195, #79858, #51203, .T. ) ;
#54308=AXIS2_PLACEMENT_3D ( 'NONE', #56676, #77827, #69313 ) ;
#54330=CARTESIAN_POINT ( 'NONE',  ( -24.99999999999999645, -19.99999999999999645, 0.000000000000000000 ) ) ;
#54468=EDGE_CURVE ( 'NONE', #60949, #33215, #9275, .T. ) ;
#54494=DIRECTION ( 'NONE',  ( -1.000000000000000000, -1.734723475976813504E-16, 0.000000000000000000 ) ) ;
#54524=CARTESIAN_POINT ( 'NONE',  ( -19.99999999999996803, 15.00000000000000711, 3.000000000000000000 ) ) ;
#54583=EDGE_CURVE ( 'NONE', #81438, #14205, #25446, .T. ) ;
#54709=ORIENTED_EDGE ( 'NONE', *, *, #23274, .F. ) ;
#54742=PRESENTATION_STYLE_ASSIGNMENT (( #82229 ) ) ;
#54955=CARTESIAN_POINT ( 'NONE',  ( 22.00000000000001066, -9.999999999999957367, 13.00000000000000178 ) ) ;
#55110=ORIENTED_EDGE ( 'NONE', *, *, #20454, .F. ) ;
#55130=( GEOMETRIC_REPRESENTATION_CONTEXT ( 3 ) GLOBAL_UNCERTAINTY_ASSIGNED_CONTEXT ( ( #83045 ) ) GLOBAL_UNIT_ASSIGNED_CONTEXT ( ( #75908, #5674, #61496 ) ) REPRESENTATION_CONTEXT ( 'NONE', 'WORKASPACE' ) );
#55133=ORIENTED_EDGE ( 'NONE', *, *, #18466, .T. ) ;
#55222=AXIS2_PLACEMENT_3D ( 'NONE', #80346, #18192, #30801 ) ;
#55281=ORIENTED_EDGE ( 'NONE', *, *, #22249, .F. ) ;
#55343=FACE_OUTER_BOUND ( 'NONE', #31919, .T. ) ;
#55375=ORIENTED_EDGE ( 'NONE', *, *, #14604, .F. ) ;
#55433=EDGE_CURVE ( 'NONE', #31499, #63487, #48930, .T. ) ;
#55545=CARTESIAN_POINT ( 'NONE',  ( -30.00000000000000000, 15.00000000000000355, 0.000000000000000000 ) ) ;
#55616=VERTEX_POINT ( 'NONE', #13271 ) ;
#55626=FACE_OUTER_BOUND ( 'NONE', #37576, .T. ) ;
#55666=AXIS2_PLACEMENT_3D ( 'NONE', #6927, #34399, #51310 ) ;
#55781=DIRECTION ( 'NONE',  ( 0.000000000000000000, 0.000000000000000000, 1.000000000000000000 ) ) ;
#55907=CARTESIAN_POINT ( 'NONE',  ( 1.653273178848927064E-15, -7.500000000000000000, 13.50000000000000178 ) ) ;
#56056=ORIENTED_EDGE ( 'NONE', *, *, #41723, .F. ) ;
#56154=DIRECTION ( 'NONE',  ( 1.000000000000000000, 0.000000000000000000, 0.000000000000000000 ) ) ;
#56188=CARTESIAN_POINT ( 'NONE',  ( -2.939152317953646711E-15, 7.500000000000000000, 13.50000000000000178 ) ) ;
#56360=VECTOR ( 'NONE', #29347, 1000.000000000000000 ) ;
#56420=VECTOR ( 'NONE', #75925, 1000.000000000000000 ) ;
#56469=( NAMED_UNIT ( * ) PLANE_ANGLE_UNIT ( ) SI_UNIT ( $, .RADIAN. ) );
#56493=ORIENTED_EDGE ( 'NONE', *, *, #83979, .F. ) ;
#56497=CARTESIAN_POINT ( 'NONE',  ( -2.939152317953646711E-15, 7.500000000000000000, 13.00000000000000178 ) ) ;
#56674=CARTESIAN_POINT ( 'NONE',  ( 1.653273178848927064E-15, -7.500000000000000000, 14.00000000000000178 ) ) ;
#56676=CARTESIAN_POINT ( 'NONE',  ( 1.653273178848927064E-15, -7.500000000000000000, 13.50000000000000178 ) ) ;
#56831=PLANE ( 'NONE',  #8784 ) ;
#56876=ORIENTED_EDGE ( 'NONE', *, *, #83979, .T. ) ;
#56884=EDGE_CURVE ( 'NONE', #2315, #18504, #69988, .T. ) ;
#56887=CARTESIAN_POINT ( 'NONE',  ( -19.99999999999996803, 15.00000000000000711, 13.00000000000000178 ) ) ;
#56899=( LENGTH_UNIT ( ) NAMED_UNIT ( * ) SI_UNIT ( .MILLI., .METRE. ) );
#56949=ORIENTED_EDGE ( 'NONE', *, *, #442, .F. ) ;
#56952=DIRECTION ( 'NONE',  ( -0.000000000000000000, -1.000000000000000000, -0.000000000000000000 ) ) ;
#57004=AXIS2_PLACEMENT_3D ( 'NONE', #66199, #75193, #68422 ) ;
#57021=CARTESIAN_POINT ( 'NONE',  ( -2.999999999999998224, -7.500000000000000000, 10.00000000000000178 ) ) ;
#57100=CARTESIAN_POINT ( 'NONE',  ( 25.00000000000000355, 9.999999999999971578, 13.00000000000000178 ) ) ;
#57281=ORIENTED_EDGE ( 'NONE', *, *, #74036, .T. ) ;
#57313=DIRECTION ( 'NONE',  ( -1.000000000000000000, 0.000000000000000000, 0.000000000000000000 ) ) ;
#57352=DIRECTION ( 'NONE',  ( 1.000000000000000000, 1.734723475976812518E-16, -0.000000000000000000 ) ) ;
#57378=EDGE_CURVE ( 'NONE', #20400, #68350, #83857, .T. ) ;
#57434=CYLINDRICAL_SURFACE ( 'NONE', #80631, 2.000000000000001776 ) ;
#57548=LINE ( 'NONE', #30086, #83001 ) ;
#57558=DIRECTION ( 'NONE',  ( 1.000000000000000000, 0.000000000000000000, 0.000000000000000000 ) ) ;
#57602=AXIS2_PLACEMENT_3D ( 'NONE', #56674, #55781, #35970 ) ;
#57647=DIRECTION ( 'NONE',  ( -1.000000000000000000, 0.000000000000000000, 0.000000000000000000 ) ) ;
#57730=CIRCLE ( 'NONE', #67776, 1.999999999999998224 ) ;
#57793=ORIENTED_EDGE ( 'NONE', *, *, #78408, .T. ) ;
#57813=PRODUCT_DEFINITION_SHAPE ( 'NONE', 'NONE',  #79883 ) ;
#57818=DIRECTION ( 'NONE',  ( 1.000000000000000000, 0.000000000000000000, 0.000000000000000000 ) ) ;
#57893=CARTESIAN_POINT ( 'NONE',  ( -2.939152317953646711E-15, 7.500000000000000000, 13.50000000000000178 ) ) ;
#57898=VECTOR ( 'NONE', #14708, 1000.000000000000000 ) ;
#57944=COLOUR_RGB ( '', 0.08235294, 0.09019608, 0.10196078) ;
#58047=CARTESIAN_POINT ( 'NONE',  ( -4.500000000000003553, 7.499999999999996447, 13.50000000000000178 ) ) ;
#58064=LINE ( 'NONE', #38247, #22769 ) ;
#58155=EDGE_CURVE ( 'NONE', #17681, #36898, #15170, .T. ) ;
#58159=AXIS2_PLACEMENT_3D ( 'NONE', #88908, #88032, #82586 ) ;
#58160=DIRECTION ( 'NONE',  ( -1.000000000000000000, 0.000000000000000000, 0.000000000000000000 ) ) ;
#58290=AXIS2_PLACEMENT_3D ( 'NONE', #44218, #24403, #57313 ) ;
#58388=CARTESIAN_POINT ( 'NONE',  ( -24.99999999999999645, 12.00000000000000711, 0.000000000000000000 ) ) ;
#58467=ORIENTED_EDGE ( 'NONE', *, *, #73665, .F. ) ;
#58774=CARTESIAN_POINT ( 'NONE',  ( -2.999999999999998224, -7.500000000000000000, 14.00000000000000178 ) ) ;
#58845=LINE ( 'NONE', #3456, #15637 ) ;
#58861=VECTOR ( 'NONE', #87914, 1000.000000000000000 ) ;
#58914=AXIS2_PLACEMENT_3D ( 'NONE', #11113, #11567, #86802 ) ;
#58998=VECTOR ( 'NONE', #61648, 1000.000000000000000 ) ;
#59151=DIRECTION ( 'NONE',  ( 0.000000000000000000, 0.000000000000000000, 1.000000000000000000 ) ) ;
#59176=CARTESIAN_POINT ( 'NONE',  ( 4.499999999999999112, 7.500000000000002665, 13.00000000000000178 ) ) ;
#59290=DIRECTION ( 'NONE',  ( -1.000000000000000000, 0.000000000000000000, 0.000000000000000000 ) ) ;
#59343=DIRECTION ( 'NONE',  ( 1.000000000000000000, 0.000000000000000000, 0.000000000000000000 ) ) ;
#59406=ORIENTED_EDGE ( 'NONE', *, *, #10571, .T. ) ;
#59441=AXIS2_PLACEMENT_3D ( 'NONE', #64701, #30483, #71461 ) ;
#59616=VERTEX_POINT ( 'NONE', #24032 ) ;
#59617=CARTESIAN_POINT ( 'NONE',  ( 3.999999999999997335, 7.500000000000000888, 14.00000000000000178 ) ) ;
#59620=CARTESIAN_POINT ( 'NONE',  ( -30.00000000000000000, -15.00000000000000000, 3.000000000000000000 ) ) ;
#59642=CARTESIAN_POINT ( 'NONE',  ( 20.00000000000000711, -9.999999999999994671, 10.00000000000000178 ) ) ;
#59692=CARTESIAN_POINT ( 'NONE',  ( -25.00000000000000355, 9.999999999999971578, 13.00000000000000178 ) ) ;
#59777=ORIENTED_EDGE ( 'NONE', *, *, #76165, .T. ) ;
#59789=CARTESIAN_POINT ( 'NONE',  ( -19.99999999999996447, -15.00000000000000533, 3.000000000000000000 ) ) ;
#59835=CARTESIAN_POINT ( 'NONE',  ( 20.00000000000000711, -9.999999999999994671, 13.00000000000000178 ) ) ;
#59884=CARTESIAN_POINT ( 'NONE',  ( -4.500000000000003553, 7.499999999999996447, 13.00000000000000178 ) ) ;
#59910=AXIS2_PLACEMENT_3D ( 'NONE', #70432, #57352, #84397 ) ;
#59914=ORIENTED_EDGE ( 'NONE', *, *, #56884, .T. ) ;
#60003=CARTESIAN_POINT ( 'NONE',  ( -22.00000000000000711, 9.999999999999971578, 10.00000000000000178 ) ) ;
#60089=EDGE_LOOP ( 'NONE', ( #43347, #71765, #59777, #63703 ) ) ;
#60171=DIRECTION ( 'NONE',  ( -0.000000000000000000, -0.000000000000000000, 1.000000000000000000 ) ) ;
#60206=DIRECTION ( 'NONE',  ( -1.000000000000000000, -2.602085213965214586E-16, 0.000000000000000000 ) ) ;
#60271=DIRECTION ( 'NONE',  ( -0.000000000000000000, -0.000000000000000000, -1.000000000000000000 ) ) ;
#60368=FACE_OUTER_BOUND ( 'NONE', #74907, .T. ) ;
#60372=VERTEX_POINT ( 'NONE', #6523 ) ;
#60379=CARTESIAN_POINT ( 'NONE',  ( -19.99999999999996447, -15.00000000000000533, 13.00000000000000178 ) ) ;
#60476=EDGE_CURVE ( 'NONE', #63332, #18616, #35070, .T. ) ;
#60639=VERTEX_POINT ( 'NONE', #85724 ) ;
#60649=DIRECTION ( 'NONE',  ( -2.602085213965214586E-16, 1.000000000000000000, 0.000000000000000000 ) ) ;
#60723=DIRECTION ( 'NONE',  ( 0.000000000000000000, 0.000000000000000000, 1.000000000000000000 ) ) ;
#60734=EDGE_CURVE ( 'NONE', #8309, #68985, #22498, .T. ) ;
#60844=PLANE ( 'NONE',  #73271 ) ;
#60867=CARTESIAN_POINT ( 'NONE',  ( -4.000000000000002665, 7.500000000000000000, 13.50000000000000178 ) ) ;
#60934=ORIENTED_EDGE ( 'NONE', *, *, #5496, .F. ) ;
#60949=VERTEX_POINT ( 'NONE', #62478 ) ;
#60977=CARTESIAN_POINT ( 'NONE',  ( -2.939152317953646711E-15, 7.500000000000000000, 13.50000000000000178 ) ) ;
#61070=FACE_OUTER_BOUND ( 'NONE', #38639, .T. ) ;
#61209=LINE ( 'NONE', #41847, #69879 ) ;
#61276=ORIENTED_EDGE ( 'NONE', *, *, #22871, .F. ) ;
#61389=ORIENTED_EDGE ( 'NONE', *, *, #55433, .F. ) ;
#61417=VERTEX_POINT ( 'NONE', #55545 ) ;
#61420=CYLINDRICAL_SURFACE ( 'NONE', #55666, 5.000000000000000888 ) ;
#61452=ORIENTED_EDGE ( 'NONE', *, *, #11703, .T. ) ;
#61496=( NAMED_UNIT ( * ) SI_UNIT ( $, .STERADIAN. ) SOLID_ANGLE_UNIT ( ) );
#61564=CARTESIAN_POINT ( 'NONE',  ( 20.00000000000000355, 10.00000000000000533, 13.00000000000000178 ) ) ;
#61566=CARTESIAN_POINT ( 'NONE',  ( 25.00000000000000355, 9.999999999999971578, 3.000000000000000000 ) ) ;
#61609=DIRECTION ( 'NONE',  ( 0.000000000000000000, -1.000000000000000000, 0.000000000000000000 ) ) ;
#61648=DIRECTION ( 'NONE',  ( -0.000000000000000000, -0.000000000000000000, -1.000000000000000000 ) ) ;
#61739=DIRECTION ( 'NONE',  ( 0.000000000000000000, -1.000000000000000000, 0.000000000000000000 ) ) ;
#61758=AXIS2_PLACEMENT_3D ( 'NONE', #76102, #88760, #75657 ) ;
#61786=ORIENTED_EDGE ( 'NONE', *, *, #18530, .F. ) ;
#61822=DIRECTION ( 'NONE',  ( -1.000000000000000000, 0.000000000000000000, 0.000000000000000000 ) ) ;
#61944=CARTESIAN_POINT ( 'NONE',  ( -24.99999999999999645, -19.99999999999999645, 3.000000000000000000 ) ) ;
#62244=DIRECTION ( 'NONE',  ( 1.000000000000000000, 0.000000000000000000, 0.000000000000000000 ) ) ;
#62373=EDGE_CURVE ( 'NONE', #61417, #34053, #28094, .T. ) ;
#62419=CARTESIAN_POINT ( 'NONE',  ( 24.99999999999999645, 20.00000000000000355, 3.000000000000000000 ) ) ;
#62427=VERTEX_POINT ( 'NONE', #80677 ) ;
#62452=FACE_OUTER_BOUND ( 'NONE', #82069, .T. ) ;
#62478=CARTESIAN_POINT ( 'NONE',  ( -4.500000000000000000, -7.499999999999999112, 13.50000000000000178 ) ) ;
#62548=ORIENTED_EDGE ( 'NONE', *, *, #67902, .F. ) ;
#62564=ORIENTED_EDGE ( 'NONE', *, *, #47035, .T. ) ;
#62617=ORIENTED_EDGE ( 'NONE', *, *, #76165, .F. ) ;
#62657=DIRECTION ( 'NONE',  ( 1.000000000000000000, 0.000000000000000000, 0.000000000000000000 ) ) ;
#62763=CARTESIAN_POINT ( 'NONE',  ( 0.000000000000000000, 0.000000000000000000, 0.000000000000000000 ) ) ;
#62823=LINE ( 'NONE', #21857, #8402 ) ;
#62884=ORIENTED_EDGE ( 'NONE', *, *, #8086, .T. ) ;
#62940=DIRECTION ( 'NONE',  ( 0.000000000000000000, 0.000000000000000000, 1.000000000000000000 ) ) ;
#63098=ORIENTED_EDGE ( 'NONE', *, *, #8218, .F. ) ;
#63214=SURFACE_SIDE_STYLE ('',( #76744 ) ) ;
#63228=ADVANCED_FACE ( 'NONE', ( #44443 ), #78243, .T. ) ;
#63332=VERTEX_POINT ( 'NONE', #66057 ) ;
#63339=DIRECTION ( 'NONE',  ( 1.734723475976812518E-16, -1.000000000000000000, 0.000000000000000000 ) ) ;
#63348=DIRECTION ( 'NONE',  ( 0.000000000000000000, 0.000000000000000000, -1.000000000000000000 ) ) ;
#63487=VERTEX_POINT ( 'NONE', #35389 ) ;
#63577=CARTESIAN_POINT ( 'NONE',  ( -2.939152317953646711E-15, 7.500000000000000000, 0.000000000000000000 ) ) ;
#63703=ORIENTED_EDGE ( 'NONE', *, *, #27715, .T. ) ;
#63737=STYLED_ITEM ( 'NONE', ( #54742 ), #28450 ) ;
#63749=VECTOR ( 'NONE', #83527, 1000.000000000000000 ) ;
#63766=DIRECTION ( 'NONE',  ( -1.000000000000000000, 0.000000000000000000, 0.000000000000000000 ) ) ;
#63778=CYLINDRICAL_SURFACE ( 'NONE', #84444, 5.000000000000000888 ) ;
#63806=FACE_OUTER_BOUND ( 'NONE', #3768, .T. ) ;
#63835=ADVANCED_FACE ( 'NONE', ( #33956 ), #61420, .T. ) ;
#64094=CARTESIAN_POINT ( 'NONE',  ( 19.99999999999997158, -14.99999999999999467, 13.00000000000000178 ) ) ;
#64186=EDGE_CURVE ( 'NONE', #53590, #17102, #57548, .T. ) ;
#64258=CARTESIAN_POINT ( 'NONE',  ( 20.00000000000000355, 10.00000000000000533, 10.00000000000000178 ) ) ;
#64291=CARTESIAN_POINT ( 'NONE',  ( 22.00000000000001066, -14.99999999999999112, 0.000000000000000000 ) ) ;
#64292=CARTESIAN_POINT ( 'NONE',  ( 25.00000000000000355, 9.999999999999971578, 13.00000000000000178 ) ) ;
#64379=VECTOR ( 'NONE', #38920, 1000.000000000000000 ) ;
#64434=EDGE_CURVE ( 'NONE', #60949, #31499, #38441, .T. ) ;
#64470=VERTEX_POINT ( 'NONE', #62419 ) ;
#64655=DIRECTION ( 'NONE',  ( -1.000000000000000000, 0.000000000000000000, 0.000000000000000000 ) ) ;
#64701=CARTESIAN_POINT ( 'NONE',  ( -24.99999999999999645, -15.00000000000000000, 3.000000000000000000 ) ) ;
#64753=LINE ( 'NONE', #22894, #15953 ) ;
#64801=ORIENTED_EDGE ( 'NONE', *, *, #28372, .F. ) ;
#64894=AXIS2_PLACEMENT_3D ( 'NONE', #63577, #557, #62244 ) ;
#64941=ORIENTED_EDGE ( 'NONE', *, *, #39224, .F. ) ;
#65063=CARTESIAN_POINT ( 'NONE',  ( -19.99999999999996447, -12.00000000000000355, 10.00000000000000178 ) ) ;
#65222=CYLINDRICAL_SURFACE ( 'NONE', #50125, 1.999999999999998224 ) ;
#65340=AXIS2_PLACEMENT_3D ( 'NONE', #29241, #77413, #36433 ) ;
#65396=CYLINDRICAL_SURFACE ( 'NONE', #58290, 5.000000000000000888 ) ;
#65535=ORIENTED_EDGE ( 'NONE', *, *, #442, .T. ) ;
#65557=EDGE_CURVE ( 'NONE', #67458, #2192, #81020, .T. ) ;
#65589=SURFACE_SIDE_STYLE ('',( #38130 ) ) ;
#65611=DIRECTION ( 'NONE',  ( 1.000000000000000000, 0.000000000000000000, 0.000000000000000000 ) ) ;
#65643=CARTESIAN_POINT ( 'NONE',  ( 1.653273178848927064E-15, -7.500000000000000000, 0.000000000000000000 ) ) ;
#65699=CARTESIAN_POINT ( 'NONE',  ( 19.99999999999996803, 12.00000000000000711, 0.000000000000000000 ) ) ;
#65843=DIRECTION ( 'NONE',  ( 1.000000000000000000, 0.000000000000000000, 0.000000000000000000 ) ) ;
#65851=LINE ( 'NONE', #24871, #54043 ) ;
#65974=ADVANCED_FACE ( 'NONE', ( #63806 ), #30031, .T. ) ;
#65987=ORIENTED_EDGE ( 'NONE', *, *, #312, .T. ) ;
#66057=CARTESIAN_POINT ( 'NONE',  ( 3.000000000000001776, -7.500000000000000000, 10.00000000000000178 ) ) ;
#66099=VECTOR ( 'NONE', #52646, 1000.000000000000000 ) ;
#66199=CARTESIAN_POINT ( 'NONE',  ( -24.99999999999999645, -15.00000000000000000, 3.000000000000000000 ) ) ;
#66223=ORIENTED_EDGE ( 'NONE', *, *, #42003, .F. ) ;
#66233=EDGE_CURVE ( 'NONE', #38114, #30359, #37931, .T. ) ;
#66238=VECTOR ( 'NONE', #27400, 1000.000000000000000 ) ;
#66299=DIRECTION ( 'NONE',  ( 0.000000000000000000, 0.000000000000000000, 1.000000000000000000 ) ) ;
#66453=CARTESIAN_POINT ( 'NONE',  ( -24.99999999999999645, -19.99999999999999645, 3.000000000000000000 ) ) ;
#66682=CARTESIAN_POINT ( 'NONE',  ( 1.653273178848927064E-15, -7.500000000000000000, 14.00000000000000178 ) ) ;
#66763=LINE ( 'NONE', #60003, #23924 ) ;
#66801=CARTESIAN_POINT ( 'NONE',  ( -22.00000000000000355, -10.00000000000000533, 13.00000000000000178 ) ) ;
#66812=VERTEX_POINT ( 'NONE', #75677 ) ;
#66863=ORIENTED_EDGE ( 'NONE', *, *, #42003, .T. ) ;
#67005=DIRECTION ( 'NONE',  ( -0.000000000000000000, -0.000000000000000000, -1.000000000000000000 ) ) ;
#67071=DIRECTION ( 'NONE',  ( -1.000000000000000000, 0.000000000000000000, 0.000000000000000000 ) ) ;
#67175=CARTESIAN_POINT ( 'NONE',  ( 20.00000000000000711, -9.999999999999994671, 3.000000000000000000 ) ) ;
#67225=CARTESIAN_POINT ( 'NONE',  ( 22.00000000000001066, -9.999999999999957367, 10.00000000000000178 ) ) ;
#67363=EDGE_CURVE ( 'NONE', #84614, #64470, #29386, .T. ) ;
#67458=VERTEX_POINT ( 'NONE', #16324 ) ;
#67592=DIRECTION ( 'NONE',  ( 1.000000000000000000, 2.602085213965214586E-16, 0.000000000000000000 ) ) ;
#67612=CARTESIAN_POINT ( 'NONE',  ( -25.00000000000000355, 9.999999999999971578, 13.00000000000000178 ) ) ;
#67631=COLOUR_RGB ( '', 0.08235294, 0.09019608, 0.10196078) ;
#67736=DIRECTION ( 'NONE',  ( -1.734723475976813504E-16, 1.000000000000000000, 0.000000000000000000 ) ) ;
#67776=AXIS2_PLACEMENT_3D ( 'NONE', #25792, #80751, #46934 ) ;
#67902=EDGE_CURVE ( 'NONE', #85628, #26549, #3577, .T. ) ;
#68168=DIRECTION ( 'NONE',  ( -0.000000000000000000, -0.000000000000000000, 1.000000000000000000 ) ) ;
#68181=DIRECTION ( 'NONE',  ( -0.000000000000000000, -0.000000000000000000, -1.000000000000000000 ) ) ;
#68185=CIRCLE ( 'NONE', #73901, 4.500000000000001776 ) ;
#68239=AXIS2_PLACEMENT_3D ( 'NONE', #9211, #8320, #83988 ) ;
#68350=VERTEX_POINT ( 'NONE', #25534 ) ;
#68422=DIRECTION ( 'NONE',  ( -1.000000000000000000, 0.000000000000000000, 0.000000000000000000 ) ) ;
#68495=VECTOR ( 'NONE', #78664, 1000.000000000000000 ) ;
#68542=EDGE_LOOP ( 'NONE', ( #57281, #46084, #88994, #12639, #45737, #33997, #20468, #13266 ) ) ;
#68570=ADVANCED_FACE ( 'NONE', ( #80273 ), #11358, .F. ) ;
#68582=EDGE_CURVE ( 'NONE', #70011, #68729, #19407, .T. ) ;
#68591=AXIS2_PLACEMENT_3D ( 'NONE', #35857, #48025, #6609 ) ;
#68729=VERTEX_POINT ( 'NONE', #31918 ) ;
#68762=AXIS2_PLACEMENT_3D ( 'NONE', #69755, #7173, #83730 ) ;
#68787=FACE_BOUND ( 'NONE', #5413, .T. ) ;
#68883=ORIENTED_EDGE ( 'NONE', *, *, #42792, .F. ) ;
#68903=AXIS2_PLACEMENT_3D ( 'NONE', #52527, #60171, #87675 ) ;
#68925=ADVANCED_FACE ( 'NONE', ( #37933 ), #65396, .T. ) ;
#68935=EDGE_LOOP ( 'NONE', ( #21358, #83699, #16150, #26585, #19919, #23800, #61452, #33418 ) ) ;
#68985=VERTEX_POINT ( 'NONE', #79364 ) ;
#69030=( GEOMETRIC_REPRESENTATION_CONTEXT ( 3 ) GLOBAL_UNCERTAINTY_ASSIGNED_CONTEXT ( ( #43713 ) ) GLOBAL_UNIT_ASSIGNED_CONTEXT ( ( #56899, #42081, #77623 ) ) REPRESENTATION_CONTEXT ( 'NONE', 'WORKASPACE' ) );
#69239=EDGE_LOOP ( 'NONE', ( #5519, #17976 ) ) ;
#69313=DIRECTION ( 'NONE',  ( -1.000000000000000000, 0.000000000000000000, 0.000000000000000000 ) ) ;
#69348=CIRCLE ( 'NONE', #29113, 2.000000000000001776 ) ;
#69504=CARTESIAN_POINT ( 'NONE',  ( -4.500000000000003553, 7.499999999999996447, 13.50000000000000178 ) ) ;
#69698=EDGE_LOOP ( 'NONE', ( #51417, #30553, #34095, #66863 ) ) ;
#69709=AXIS2_PLACEMENT_3D ( 'NONE', #51163, #71025, #29604 ) ;
#69755=CARTESIAN_POINT ( 'NONE',  ( -2.939152317953646711E-15, 7.500000000000000000, 0.000000000000000000 ) ) ;
#69784=VECTOR ( 'NONE', #79647, 1000.000000000000000 ) ;
#69789=DIRECTION ( 'NONE',  ( -0.000000000000000000, -0.000000000000000000, -1.000000000000000000 ) ) ;
#69879=VECTOR ( 'NONE', #76510, 1000.000000000000000 ) ;
#69988=LINE ( 'NONE', #35779, #63749 ) ;
#69990=AXIS2_PLACEMENT_3D ( 'NONE', #49808, #8840, #63766 ) ;
#69999=VERTEX_POINT ( 'NONE', #23655 ) ;
#70011=VERTEX_POINT ( 'NONE', #58774 ) ;
#70389=CARTESIAN_POINT ( 'NONE',  ( -3.999999999999998224, -7.500000000000000000, 13.50000000000000178 ) ) ;
#70432=CARTESIAN_POINT ( 'NONE',  ( -22.00000000000000711, 9.999999999999971578, 13.00000000000000178 ) ) ;
#70435=EDGE_CURVE ( 'NONE', #67458, #79858, #61209, .T. ) ;
#70518=AXIS2_PLACEMENT_3D ( 'NONE', #31813, #39465, #32256 ) ;
#70560=AXIS2_PLACEMENT_3D ( 'NONE', #17344, #44802, #72281 ) ;
#70571=CARTESIAN_POINT ( 'NONE',  ( 20.00000000000000355, 10.00000000000000533, 0.000000000000000000 ) ) ;
#70584=LINE ( 'NONE', #42675, #13026 ) ;
#70876=FILL_AREA_STYLE_COLOUR ( '', #67631 ) ;
#70886=CIRCLE ( 'NONE', #82410, 4.000000000000000000 ) ;
#70974=DIRECTION ( 'NONE',  ( -1.000000000000000000, 0.000000000000000000, 0.000000000000000000 ) ) ;
#71025=DIRECTION ( 'NONE',  ( 0.000000000000000000, 0.000000000000000000, 1.000000000000000000 ) ) ;
#71058=DIRECTION ( 'NONE',  ( -1.000000000000000000, -1.734723475976813504E-16, 0.000000000000000000 ) ) ;
#71125=ORIENTED_EDGE ( 'NONE', *, *, #53106, .F. ) ;
#71148=FACE_OUTER_BOUND ( 'NONE', #30457, .T. ) ;
#71194=EDGE_LOOP ( 'NONE', ( #75806, #7893, #31447, #75673 ) ) ;
#71278=CARTESIAN_POINT ( 'NONE',  ( 2.999999999999997335, 7.500000000000000000, 10.00000000000000178 ) ) ;
#71296=( NAMED_UNIT ( * ) SI_UNIT ( $, .STERADIAN. ) SOLID_ANGLE_UNIT ( ) );
#71324=CARTESIAN_POINT ( 'NONE',  ( -19.99999999999996447, -15.00000000000000533, 13.00000000000000178 ) ) ;
#71363=DIRECTION ( 'NONE',  ( -0.000000000000000000, -0.000000000000000000, -1.000000000000000000 ) ) ;
#71367=CARTESIAN_POINT ( 'NONE',  ( 4.499999999999999112, 7.500000000000002665, 13.50000000000000178 ) ) ;
#71386=LINE ( 'NONE', #43922, #44377 ) ;
#71412=ADVANCED_FACE ( 'NONE', ( #8737 ), #42082, .T. ) ;
#71461=DIRECTION ( 'NONE',  ( -1.000000000000000000, 0.000000000000000000, 0.000000000000000000 ) ) ;
#71501=DIRECTION ( 'NONE',  ( 0.000000000000000000, -0.000000000000000000, -1.000000000000000000 ) ) ;
#71559=DIRECTION ( 'NONE',  ( -0.000000000000000000, -0.000000000000000000, -1.000000000000000000 ) ) ;
#71581=DIRECTION ( 'NONE',  ( 1.000000000000000000, 0.000000000000000000, 0.000000000000000000 ) ) ;
#71594=CIRCLE ( 'NONE', #83120, 4.000000000000000000 ) ;
#71705=VERTEX_POINT ( 'NONE', #67225 ) ;
#71765=ORIENTED_EDGE ( 'NONE', *, *, #9660, .F. ) ;
#71773=VECTOR ( 'NONE', #39955, 1000.000000000000000 ) ;
#71790=ORIENTED_EDGE ( 'NONE', *, *, #66233, .T. ) ;
#71849=VECTOR ( 'NONE', #39605, 1000.000000000000000 ) ;
#71913=DIRECTION ( 'NONE',  ( 0.000000000000000000, 0.000000000000000000, 1.000000000000000000 ) ) ;
#71950=DIRECTION ( 'NONE',  ( -0.000000000000000000, -0.000000000000000000, -1.000000000000000000 ) ) ;
#72025=CARTESIAN_POINT ( 'NONE',  ( -4.500000000000003553, 7.499999999999996447, 13.50000000000000178 ) ) ;
#72103=VECTOR ( 'NONE', #23749, 1000.000000000000000 ) ;
#72281=DIRECTION ( 'NONE',  ( -1.000000000000000000, 0.000000000000000000, 0.000000000000000000 ) ) ;
#72353=FILL_AREA_STYLE_COLOUR ( '', #57944 ) ;
#72370=ORIENTED_EDGE ( 'NONE', *, *, #57378, .T. ) ;
#72424=DIRECTION ( 'NONE',  ( -0.000000000000000000, -0.000000000000000000, -1.000000000000000000 ) ) ;
#72595=DIRECTION ( 'NONE',  ( 0.000000000000000000, 0.000000000000000000, 1.000000000000000000 ) ) ;
#72988=CIRCLE ( 'NONE', #31251, 4.999999999999997335 ) ;
#72990=ORIENTED_EDGE ( 'NONE', *, *, #84681, .F. ) ;
#73011=CIRCLE ( 'NONE', #6853, 5.000000000000000888 ) ;
#73020=ORIENTED_EDGE ( 'NONE', *, *, #1205, .T. ) ;
#73049=EDGE_LOOP ( 'NONE', ( #55133, #36090 ) ) ;
#73074=DIRECTION ( 'NONE',  ( 0.000000000000000000, 0.000000000000000000, 1.000000000000000000 ) ) ;
#73172=EDGE_LOOP ( 'NONE', ( #24941, #24800, #29654, #76218 ) ) ;
#73191=CARTESIAN_POINT ( 'NONE',  ( -19.99999999999996447, -15.00000000000000533, 13.00000000000000178 ) ) ;
#73271=AXIS2_PLACEMENT_3D ( 'NONE', #67612, #40151, #33385 ) ;
#73290=ADVANCED_FACE ( 'NONE', ( #50332 ), #24197, .F. ) ;
#73385=ADVANCED_FACE ( 'NONE', ( #86828 ), #31862, .T. ) ;
#73416=AXIS2_PLACEMENT_3D ( 'NONE', #10596, #78597, #16900 ) ;
#73429=ORIENTED_EDGE ( 'NONE', *, *, #7303, .T. ) ;
#73431=ORIENTED_EDGE ( 'NONE', *, *, #10571, .F. ) ;
#73452=ORIENTED_EDGE ( 'NONE', *, *, #8964, .F. ) ;
#73496=VERTEX_POINT ( 'NONE', #71278 ) ;
#73611=ADVANCED_FACE ( 'NONE', ( #24419 ), #79383, .T. ) ;
#73627=FACE_BOUND ( 'NONE', #47183, .T. ) ;
#73628=DIRECTION ( 'NONE',  ( 1.000000000000000000, 0.000000000000000000, 0.000000000000000000 ) ) ;
#73665=EDGE_CURVE ( 'NONE', #17102, #18504, #65851, .T. ) ;
#73804=LINE ( 'NONE', #24711, #16889 ) ;
#73851=DIRECTION ( 'NONE',  ( -0.000000000000000000, -0.000000000000000000, -1.000000000000000000 ) ) ;
#73901=AXIS2_PLACEMENT_3D ( 'NONE', #79436, #59151, #86203 ) ;
#73906=AXIS2_PLACEMENT_3D ( 'NONE', #65643, #53020, #59343 ) ;
#73937=DIRECTION ( 'NONE',  ( 1.000000000000000000, 0.000000000000000000, 0.000000000000000000 ) ) ;
#73979=AXIS2_PLACEMENT_3D ( 'NONE', #15496, #10051, #29022 ) ;
#73996=ADVANCED_BREP_SHAPE_REPRESENTATION ( '', ( #28450, #83448 ), #69030 ) ;
#74036=EDGE_CURVE ( 'NONE', #33584, #3413, #6665, .T. ) ;
#74100=ORIENTED_EDGE ( 'NONE', *, *, #1306, .T. ) ;
#74270=ORIENTED_EDGE ( 'NONE', *, *, #26808, .T. ) ;
#74345=LINE ( 'NONE', #54955, #5110 ) ;
#74381=CARTESIAN_POINT ( 'NONE',  ( -2.939152317953646711E-15, 7.500000000000000000, 14.00000000000000178 ) ) ;
#74585=DIRECTION ( 'NONE',  ( 0.000000000000000000, -0.000000000000000000, -1.000000000000000000 ) ) ;
#74626=ORIENTED_EDGE ( 'NONE', *, *, #984, .F. ) ;
#74658=ADVANCED_FACE ( 'NONE', ( #3841 ), #86287, .T. ) ;
#74667=EDGE_LOOP ( 'NONE', ( #27672, #87569, #46019, #11811 ) ) ;
#74786=DIRECTION ( 'NONE',  ( 1.734723475976813504E-16, -1.000000000000000000, 0.000000000000000000 ) ) ;
#74895=ORIENTED_EDGE ( 'NONE', *, *, #42626, .F. ) ;
#74907=EDGE_LOOP ( 'NONE', ( #83097, #55110, #34993, #14744 ) ) ;
#75005=PLANE ( 'NONE',  #7746 ) ;
#75066=LINE ( 'NONE', #75941, #13006 ) ;
#75193=DIRECTION ( 'NONE',  ( 0.000000000000000000, 0.000000000000000000, 1.000000000000000000 ) ) ;
#75538=PLANE ( 'NONE',  #81236 ) ;
#75654=ORIENTED_EDGE ( 'NONE', *, *, #41283, .F. ) ;
#75657=DIRECTION ( 'NONE',  ( -1.000000000000000000, 0.000000000000000000, 0.000000000000000000 ) ) ;
#75673=ORIENTED_EDGE ( 'NONE', *, *, #8218, .T. ) ;
#75677=CARTESIAN_POINT ( 'NONE',  ( -24.99999999999999645, 20.00000000000000355, 0.000000000000000000 ) ) ;
#75754=CIRCLE ( 'NONE', #36862, 3.000000000000000000 ) ;
#75759=EDGE_CURVE ( 'NONE', #53590, #2315, #73804, .T. ) ;
#75789=CARTESIAN_POINT ( 'NONE',  ( -24.99999999999999645, -12.00000000000000533, 0.000000000000000000 ) ) ;
#75806=ORIENTED_EDGE ( 'NONE', *, *, #11703, .F. ) ;
#75908=( LENGTH_UNIT ( ) NAMED_UNIT ( * ) SI_UNIT ( .MILLI., .METRE. ) );
#75925=DIRECTION ( 'NONE',  ( -1.000000000000000000, 0.000000000000000000, 0.000000000000000000 ) ) ;
#75941=CARTESIAN_POINT ( 'NONE',  ( -3.000000000000003553, 7.500000000000000000, 0.000000000000000000 ) ) ;
#76102=CARTESIAN_POINT ( 'NONE',  ( 20.00000000000000711, -9.999999999999994671, 13.00000000000000178 ) ) ;
#76118=ORIENTED_EDGE ( 'NONE', *, *, #46164, .F. ) ;
#76165=EDGE_CURVE ( 'NONE', #30359, #37043, #13752, .T. ) ;
#76181=DIRECTION ( 'NONE',  ( 0.000000000000000000, 0.000000000000000000, 1.000000000000000000 ) ) ;
#76218=ORIENTED_EDGE ( 'NONE', *, *, #84681, .T. ) ;
#76228=DIRECTION ( 'NONE',  ( 0.000000000000000000, 0.000000000000000000, 1.000000000000000000 ) ) ;
#76287=VECTOR ( 'NONE', #19664, 1000.000000000000000 ) ;
#76335=VECTOR ( 'NONE', #46985, 1000.000000000000000 ) ;
#76403=CARTESIAN_POINT ( 'NONE',  ( 4.500000000000003553, -7.499999999999999112, 13.50000000000000178 ) ) ;
#76416=EDGE_CURVE ( 'NONE', #38114, #5766, #43880, .T. ) ;
#76421=EDGE_CURVE ( 'NONE', #15649, #31320, #38501, .T. ) ;
#76492=VECTOR ( 'NONE', #31767, 1000.000000000000000 ) ;
#76510=DIRECTION ( 'NONE',  ( -0.000000000000000000, -0.000000000000000000, -1.000000000000000000 ) ) ;
#76642=VECTOR ( 'NONE', #63339, 1000.000000000000000 ) ;
#76744=SURFACE_STYLE_FILL_AREA ( #35765 ) ;
#76887=DIRECTION ( 'NONE',  ( -1.000000000000000000, -8.673617379884027583E-16, 0.000000000000000000 ) ) ;
#76916=CIRCLE ( 'NONE', #40982, 4.999999999999997335 ) ;
#77143=ORIENTED_EDGE ( 'NONE', *, *, #30623, .F. ) ;
#77321=EDGE_LOOP ( 'NONE', ( #80320, #73020 ) ) ;
#77366=DIRECTION ( 'NONE',  ( -1.000000000000000000, 0.000000000000000000, 0.000000000000000000 ) ) ;
#77394=EDGE_CURVE ( 'NONE', #4695, #22067, #62823, .T. ) ;
#77413=DIRECTION ( 'NONE',  ( 0.000000000000000000, 0.000000000000000000, 1.000000000000000000 ) ) ;
#77623=( NAMED_UNIT ( * ) SI_UNIT ( $, .STERADIAN. ) SOLID_ANGLE_UNIT ( ) );
#77650=DIRECTION ( 'NONE',  ( -0.000000000000000000, -0.000000000000000000, 1.000000000000000000 ) ) ;
#77672=ORIENTED_EDGE ( 'NONE', *, *, #30110, .T. ) ;
#77732=EDGE_LOOP ( 'NONE', ( #24232, #56056, #48965, #22215 ) ) ;
#77758=ORIENTED_EDGE ( 'NONE', *, *, #88278, .T. ) ;
#77827=DIRECTION ( 'NONE',  ( -0.000000000000000000, -0.000000000000000000, -1.000000000000000000 ) ) ;
#77939=ORIENTED_EDGE ( 'NONE', *, *, #12757, .T. ) ;
#78085=CARTESIAN_POINT ( 'NONE',  ( -3.000000000000003553, 7.500000000000000000, 14.00000000000000178 ) ) ;
#78195=CARTESIAN_POINT ( 'NONE',  ( -19.99999999999996803, 15.00000000000000711, 3.000000000000000000 ) ) ;
#78243=CYLINDRICAL_SURFACE ( 'NONE', #15377, 4.000000000000000000 ) ;
#78244=LINE ( 'NONE', #44444, #89115 ) ;
#78408=EDGE_CURVE ( 'NONE', #64470, #50943, #71386, .T. ) ;
#78481=DIRECTION ( 'NONE',  ( -0.000000000000000000, -0.000000000000000000, -1.000000000000000000 ) ) ;
#78593=DIRECTION ( 'NONE',  ( -0.000000000000000000, -0.000000000000000000, -1.000000000000000000 ) ) ;
#78597=DIRECTION ( 'NONE',  ( 0.000000000000000000, 0.000000000000000000, 1.000000000000000000 ) ) ;
#78628=ORIENTED_EDGE ( 'NONE', *, *, #26808, .F. ) ;
#78664=DIRECTION ( 'NONE',  ( -0.000000000000000000, -0.000000000000000000, -1.000000000000000000 ) ) ;
#78730=DIRECTION ( 'NONE',  ( 0.000000000000000000, 1.000000000000000000, 0.000000000000000000 ) ) ;
#78748=LINE ( 'NONE', #85514, #69784 ) ;
#78752=DIRECTION ( 'NONE',  ( 0.000000000000000000, 0.000000000000000000, 1.000000000000000000 ) ) ;
#78790=ORIENTED_EDGE ( 'NONE', *, *, #57378, .F. ) ;
#78850=ORIENTED_EDGE ( 'NONE', *, *, #18466, .F. ) ;
#78941=CLOSED_SHELL ( 'NONE', ( #73611, #49437, #53699, #29651, #33896, #9839, #28310, #33010, #4686, #74658, #14572, #68925, #28508, #4633, #48813, #50681, #73290, #63835, #37077, #17037, #22263, #65974, #49276, #48601, #8330, #47700, #28249, #42777, #71412, #24149, #73385, #85745, #46155, #3289, #31863, #63228, #25250, #48307, #32287, #43871, #85400, #43345, #68570 ) ) ;
#78963=AXIS2_PLACEMENT_3D ( 'NONE', #46854, #54494, #74786 ) ;
#79045=FACE_OUTER_BOUND ( 'NONE', #41583, .T. ) ;
#79051=CARTESIAN_POINT ( 'NONE',  ( -4.500000000000000000, -7.499999999999999112, 13.50000000000000178 ) ) ;
#79058=FACE_OUTER_BOUND ( 'NONE', #21028, .T. ) ;
#79144=DIRECTION ( 'NONE',  ( 0.000000000000000000, 0.000000000000000000, 1.000000000000000000 ) ) ;
#79199=EDGE_LOOP ( 'NONE', ( #2047, #49672, #81819, #61786, #54709, #55281, #28088, #58467 ) ) ;
#79222=CARTESIAN_POINT ( 'NONE',  ( 30.00000000000000000, 15.00000000000000355, 3.000000000000000000 ) ) ;
#79225=FACE_OUTER_BOUND ( 'NONE', #24294, .T. ) ;
#79252=DIRECTION ( 'NONE',  ( -0.000000000000000000, -0.000000000000000000, -1.000000000000000000 ) ) ;
#79293=VECTOR ( 'NONE', #31525, 1000.000000000000000 ) ;
#79364=CARTESIAN_POINT ( 'NONE',  ( -4.500000000000003553, 7.499999999999996447, 13.00000000000000178 ) ) ;
#79383=CYLINDRICAL_SURFACE ( 'NONE', #42547, 4.000000000000000000 ) ;
#79429=EDGE_LOOP ( 'NONE', ( #56949, #46610 ) ) ;
#79436=CARTESIAN_POINT ( 'NONE',  ( 1.653273178848927064E-15, -7.500000000000000000, 13.00000000000000178 ) ) ;
#79550=VERTEX_POINT ( 'NONE', #78195 ) ;
#79630=ORIENTED_EDGE ( 'NONE', *, *, #53279, .T. ) ;
#79647=DIRECTION ( 'NONE',  ( 1.734723475976812518E-16, -1.000000000000000000, 0.000000000000000000 ) ) ;
#79850=CARTESIAN_POINT ( 'NONE',  ( 30.00000000000000000, -15.00000000000000000, 3.000000000000000000 ) ) ;
#79858=VERTEX_POINT ( 'NONE', #27688 ) ;
#79883=PRODUCT_DEFINITION ( 'UNKNOWN', '', #80689, #23051 ) ;
#79901=EDGE_LOOP ( 'NONE', ( #60934, #15066, #35236, #65535 ) ) ;
#79931=EDGE_CURVE ( 'NONE', #26549, #68985, #81973, .T. ) ;
#79964=EDGE_LOOP ( 'NONE', ( #7196, #46900, #83490, #46988 ) ) ;
#80069=EDGE_CURVE ( 'NONE', #51011, #69999, #5101, .T. ) ;
#80273=FACE_OUTER_BOUND ( 'NONE', #17953, .T. ) ;
#80320=ORIENTED_EDGE ( 'NONE', *, *, #60476, .T. ) ;
#80346=CARTESIAN_POINT ( 'NONE',  ( -2.939152317953646711E-15, 7.500000000000000000, 14.00000000000000178 ) ) ;
#80470=PLANE ( 'NONE',  #80668 ) ;
#80520=CYLINDRICAL_SURFACE ( 'NONE', #73906, 3.000000000000000000 ) ;
#80540=FACE_OUTER_BOUND ( 'NONE', #11101, .T. ) ;
#80631=AXIS2_PLACEMENT_3D ( 'NONE', #29536, #85367, #23653 ) ;
#80668=AXIS2_PLACEMENT_3D ( 'NONE', #34045, #4809, #47553 ) ;
#80677=CARTESIAN_POINT ( 'NONE',  ( -19.99999999999996803, 15.00000000000000711, 13.00000000000000178 ) ) ;
#80689=PRODUCT_DEFINITION_FORMATION_WITH_SPECIFIED_SOURCE ( 'ANY', '', #31988, .NOT_KNOWN. ) ;
#80751=DIRECTION ( 'NONE',  ( 0.000000000000000000, 0.000000000000000000, 1.000000000000000000 ) ) ;
#80812=LINE ( 'NONE', #13663, #22697 ) ;
#80837=ORIENTED_EDGE ( 'NONE', *, *, #67363, .F. ) ;
#80998=CARTESIAN_POINT ( 'NONE',  ( 24.99999999999999645, 20.00000000000000355, 0.000000000000000000 ) ) ;
#81011=DIRECTION ( 'NONE',  ( 1.000000000000000000, 0.000000000000000000, -0.000000000000000000 ) ) ;
#81020=CIRCLE ( 'NONE', #10541, 2.000000000000001776 ) ;
#81205=VERTEX_POINT ( 'NONE', #13638 ) ;
#81236=AXIS2_PLACEMENT_3D ( 'NONE', #21031, #82315, #35442 ) ;
#81297=EDGE_CURVE ( 'NONE', #81205, #50943, #20238, .T. ) ;
#81438=VERTEX_POINT ( 'NONE', #472 ) ;
#81482=DIRECTION ( 'NONE',  ( -0.000000000000000000, -0.000000000000000000, -1.000000000000000000 ) ) ;
#81501=CARTESIAN_POINT ( 'NONE',  ( -25.00000000000000000, -10.00000000000000533, 13.00000000000000178 ) ) ;
#81574=LINE ( 'NONE', #54524, #58861 ) ;
#81819=ORIENTED_EDGE ( 'NONE', *, *, #34301, .F. ) ;
#81949=DIRECTION ( 'NONE',  ( 0.000000000000000000, 0.000000000000000000, 1.000000000000000000 ) ) ;
#81973=CIRCLE ( 'NONE', #9994, 4.500000000000001776 ) ;
#82069=EDGE_LOOP ( 'NONE', ( #40055, #72990, #19056, #50100 ) ) ;
#82229=SURFACE_STYLE_USAGE ( .BOTH. , #65589 ) ;
#82235=DIRECTION ( 'NONE',  ( 1.000000000000000000, 0.000000000000000000, 0.000000000000000000 ) ) ;
#82315=DIRECTION ( 'NONE',  ( 0.000000000000000000, 0.000000000000000000, 1.000000000000000000 ) ) ;
#82326=CARTESIAN_POINT ( 'NONE',  ( -22.00000000000000355, -10.00000000000000533, 10.00000000000000178 ) ) ;
#82410=AXIS2_PLACEMENT_3D ( 'NONE', #60977, #25869, #25423 ) ;
#82502=VERTEX_POINT ( 'NONE', #65699 ) ;
#82586=DIRECTION ( 'NONE',  ( -1.000000000000000000, 0.000000000000000000, 0.000000000000000000 ) ) ;
#82973=VERTEX_POINT ( 'NONE', #70389 ) ;
#83001=VECTOR ( 'NONE', #71950, 1000.000000000000000 ) ;
#83005=ORIENTED_EDGE ( 'NONE', *, *, #14083, .T. ) ;
#83045=UNCERTAINTY_MEASURE_WITH_UNIT (LENGTH_MEASURE( 1.000000000000000082E-05 ), #75908, 'distance_accuracy_value', 'NONE');
#83090=FACE_BOUND ( 'NONE', #44852, .T. ) ;
#83097=ORIENTED_EDGE ( 'NONE', *, *, #54212, .F. ) ;
#83116=PLANE ( 'NONE',  #24902 ) ;
#83120=AXIS2_PLACEMENT_3D ( 'NONE', #31399, #79144, #65611 ) ;
#83158=ORIENTED_EDGE ( 'NONE', *, *, #2087, .F. ) ;
#83266=ORIENTED_EDGE ( 'NONE', *, *, #85079, .T. ) ;
#83290=AXIS2_PLACEMENT_3D ( 'NONE', #44780, #31734, #46134 ) ;
#83307=ORIENTED_EDGE ( 'NONE', *, *, #7645, .F. ) ;
#83323=DIRECTION ( 'NONE',  ( -0.000000000000000000, -0.000000000000000000, -1.000000000000000000 ) ) ;
#83442=CIRCLE ( 'NONE', #70518, 5.000000000000000888 ) ;
#83448=AXIS2_PLACEMENT_3D ( 'NONE', #62763, #83959, #35307 ) ;
#83490=ORIENTED_EDGE ( 'NONE', *, *, #1306, .F. ) ;
#83527=DIRECTION ( 'NONE',  ( -0.000000000000000000, -0.000000000000000000, -1.000000000000000000 ) ) ;
#83538=AXIS2_PLACEMENT_3D ( 'NONE', #1176, #15146, #36308 ) ;
#83550=EDGE_CURVE ( 'NONE', #19590, #66812, #4553, .T. ) ;
#83551=ORIENTED_EDGE ( 'NONE', *, *, #76421, .T. ) ;
#83659=DIRECTION ( 'NONE',  ( 0.000000000000000000, 0.000000000000000000, 1.000000000000000000 ) ) ;
#83679=FACE_OUTER_BOUND ( 'NONE', #68542, .T. ) ;
#83699=ORIENTED_EDGE ( 'NONE', *, *, #49853, .T. ) ;
#83730=DIRECTION ( 'NONE',  ( 1.000000000000000000, 0.000000000000000000, 0.000000000000000000 ) ) ;
#83857=LINE ( 'NONE', #43730, #56360 ) ;
#83885=EDGE_LOOP ( 'NONE', ( #6641, #50469, #68883, #37978 ) ) ;
#83959=DIRECTION ( 'NONE',  ( 0.000000000000000000, 0.000000000000000000, 1.000000000000000000 ) ) ;
#83979=EDGE_CURVE ( 'NONE', #84614, #81205, #2651, .T. ) ;
#83988=DIRECTION ( 'NONE',  ( -1.000000000000000000, 0.000000000000000000, 0.000000000000000000 ) ) ;
#84164=EDGE_CURVE ( 'NONE', #38465, #31293, #70584, .T. ) ;
#84255=CARTESIAN_POINT ( 'NONE',  ( -24.99999999999999645, -15.00000000000000000, 0.000000000000000000 ) ) ;
#84319=VECTOR ( 'NONE', #67736, 1000.000000000000000 ) ;
#84397=DIRECTION ( 'NONE',  ( -1.734723475976812518E-16, 1.000000000000000000, 0.000000000000000000 ) ) ;
#84444=AXIS2_PLACEMENT_3D ( 'NONE', #84512, #16487, #64655 ) ;
#84512=CARTESIAN_POINT ( 'NONE',  ( -24.99999999999999645, 15.00000000000000355, 3.000000000000000000 ) ) ;
#84614=VERTEX_POINT ( 'NONE', #23608 ) ;
#84681=EDGE_CURVE ( 'NONE', #33584, #34053, #18653, .T. ) ;
#85019=DIRECTION ( 'NONE',  ( -0.000000000000000000, -0.000000000000000000, -1.000000000000000000 ) ) ;
#85079=EDGE_CURVE ( 'NONE', #3413, #34010, #53982, .T. ) ;
#85366=CARTESIAN_POINT ( 'NONE',  ( -3.000000000000003553, 7.500000000000000000, 10.00000000000000178 ) ) ;
#85367=DIRECTION ( 'NONE',  ( -0.000000000000000000, -0.000000000000000000, -1.000000000000000000 ) ) ;
#85400=ADVANCED_FACE ( 'NONE', ( #61070 ), #80470, .F. ) ;
#85514=CARTESIAN_POINT ( 'NONE',  ( -25.00000000000000355, 9.999999999999971578, 13.00000000000000178 ) ) ;
#85628=VERTEX_POINT ( 'NONE', #71367 ) ;
#85713=SHAPE_REPRESENTATION ( 'head base', ( #83448 ), #69030 ) ;
#85724=CARTESIAN_POINT ( 'NONE',  ( 30.00000000000000000, -15.00000000000000000, 0.000000000000000000 ) ) ;
#85745=ADVANCED_FACE ( 'NONE', ( #73627, #25420, #18674 ), #12354, .F. ) ;
#85836=ORIENTED_EDGE ( 'NONE', *, *, #88278, .F. ) ;
#85911=DIRECTION ( 'NONE',  ( 1.734723475976813504E-16, -1.000000000000000000, 0.000000000000000000 ) ) ;
#86003=AXIS2_PLACEMENT_3D ( 'NONE', #24492, #31714, #51960 ) ;
#86111=CIRCLE ( 'NONE', #14164, 1.999999999999998224 ) ;
#86203=DIRECTION ( 'NONE',  ( 1.000000000000000000, 0.000000000000000000, 0.000000000000000000 ) ) ;
#86287=CYLINDRICAL_SURFACE ( 'NONE', #69990, 5.000000000000000888 ) ;
#86309=CIRCLE ( 'NONE', #21552, 4.000000000000000000 ) ;
#86352=DIRECTION ( 'NONE',  ( -1.000000000000000000, 0.000000000000000000, 0.000000000000000000 ) ) ;
#86417=ORIENTED_EDGE ( 'NONE', *, *, #39224, .T. ) ;
#86462=LINE ( 'NONE', #72025, #66099 ) ;
#86476=VECTOR ( 'NONE', #43568, 1000.000000000000000 ) ;
#86520=CARTESIAN_POINT ( 'NONE',  ( 2.999999999999997335, 7.500000000000000000, 0.000000000000000000 ) ) ;
#86526=FACE_OUTER_BOUND ( 'NONE', #43792, .T. ) ;
#86581=ORIENTED_EDGE ( 'NONE', *, *, #8086, .F. ) ;
#86795=FACE_OUTER_BOUND ( 'NONE', #79901, .T. ) ;
#86802=DIRECTION ( 'NONE',  ( 1.000000000000000000, 0.000000000000000000, 0.000000000000000000 ) ) ;
#86828=FACE_OUTER_BOUND ( 'NONE', #71194, .T. ) ;
#86912=LINE ( 'NONE', #46787, #71849 ) ;
#87087=CARTESIAN_POINT ( 'NONE',  ( 4.500000000000003553, -7.499999999999999112, 13.50000000000000178 ) ) ;
#87142=DIRECTION ( 'NONE',  ( 1.000000000000000000, 0.000000000000000000, -0.000000000000000000 ) ) ;
#87166=AXIS2_PLACEMENT_3D ( 'NONE', #2561, #30487, #16528 ) ;
#87225=LINE ( 'NONE', #28610, #21824 ) ;
#87304=CARTESIAN_POINT ( 'NONE',  ( 20.00000000000000711, -9.999999999999994671, 13.00000000000000178 ) ) ;
#87328=DIRECTION ( 'NONE',  ( -1.734723475976813750E-16, 1.000000000000000000, -0.000000000000000000 ) ) ;
#87345=AXIS2_PLACEMENT_3D ( 'NONE', #38627, #44473, #57558 ) ;
#87475=FACE_OUTER_BOUND ( 'NONE', #88910, .T. ) ;
#87504=DIRECTION ( 'NONE',  ( 1.734723475976812518E-16, -1.000000000000000000, 0.000000000000000000 ) ) ;
#87518=AXIS2_PLACEMENT_3D ( 'NONE', #61564, #33666, #40868 ) ;
#87569=ORIENTED_EDGE ( 'NONE', *, *, #18066, .F. ) ;
#87635=AXIS2_PLACEMENT_3D ( 'NONE', #31913, #78752, #44509 ) ;
#87675=DIRECTION ( 'NONE',  ( 1.000000000000000000, 0.000000000000000000, 0.000000000000000000 ) ) ;
#87703=CIRCLE ( 'NONE', #53210, 4.000000000000000000 ) ;
#87752=ORIENTED_EDGE ( 'NONE', *, *, #38282, .F. ) ;
#87914=DIRECTION ( 'NONE',  ( -1.000000000000000000, -0.000000000000000000, -0.000000000000000000 ) ) ;
#87973=DIRECTION ( 'NONE',  ( 0.000000000000000000, 0.000000000000000000, 1.000000000000000000 ) ) ;
#88001=CARTESIAN_POINT ( 'NONE',  ( 3.999999999999997335, 7.500000000000000888, 13.50000000000000178 ) ) ;
#88032=DIRECTION ( 'NONE',  ( 0.000000000000000000, 0.000000000000000000, 1.000000000000000000 ) ) ;
#88124=ORIENTED_EDGE ( 'NONE', *, *, #77394, .F. ) ;
#88237=AXIS2_PLACEMENT_3D ( 'NONE', #50276, #2987, #30465 ) ;
#88278=EDGE_CURVE ( 'NONE', #18545, #62427, #8277, .T. ) ;
#88365=ORIENTED_EDGE ( 'NONE', *, *, #76416, .T. ) ;
#88395=APPLICATION_CONTEXT ( 'automotive_design' ) ;
#88419=AXIS2_PLACEMENT_3D ( 'NONE', #4604, #37946, #32077 ) ;
#88760=DIRECTION ( 'NONE',  ( -0.000000000000000000, -0.000000000000000000, -1.000000000000000000 ) ) ;
#88908=CARTESIAN_POINT ( 'NONE',  ( 24.99999999999999645, 15.00000000000000355, 3.000000000000000000 ) ) ;
#88910=EDGE_LOOP ( 'NONE', ( #6206, #27557, #85836, #6220 ) ) ;
#88931=ORIENTED_EDGE ( 'NONE', *, *, #14604, .T. ) ;
#88977=CARTESIAN_POINT ( 'NONE',  ( -2.939152317953646711E-15, 7.500000000000000000, 13.50000000000000178 ) ) ;
#88994=ORIENTED_EDGE ( 'NONE', *, *, #49596, .T. ) ;
#89087=FACE_OUTER_BOUND ( 'NONE', #23952, .T. ) ;
#89115=VECTOR ( 'NONE', #22857, 1000.000000000000000 ) ;
ENDSEC;
END-ISO-10303-21;
